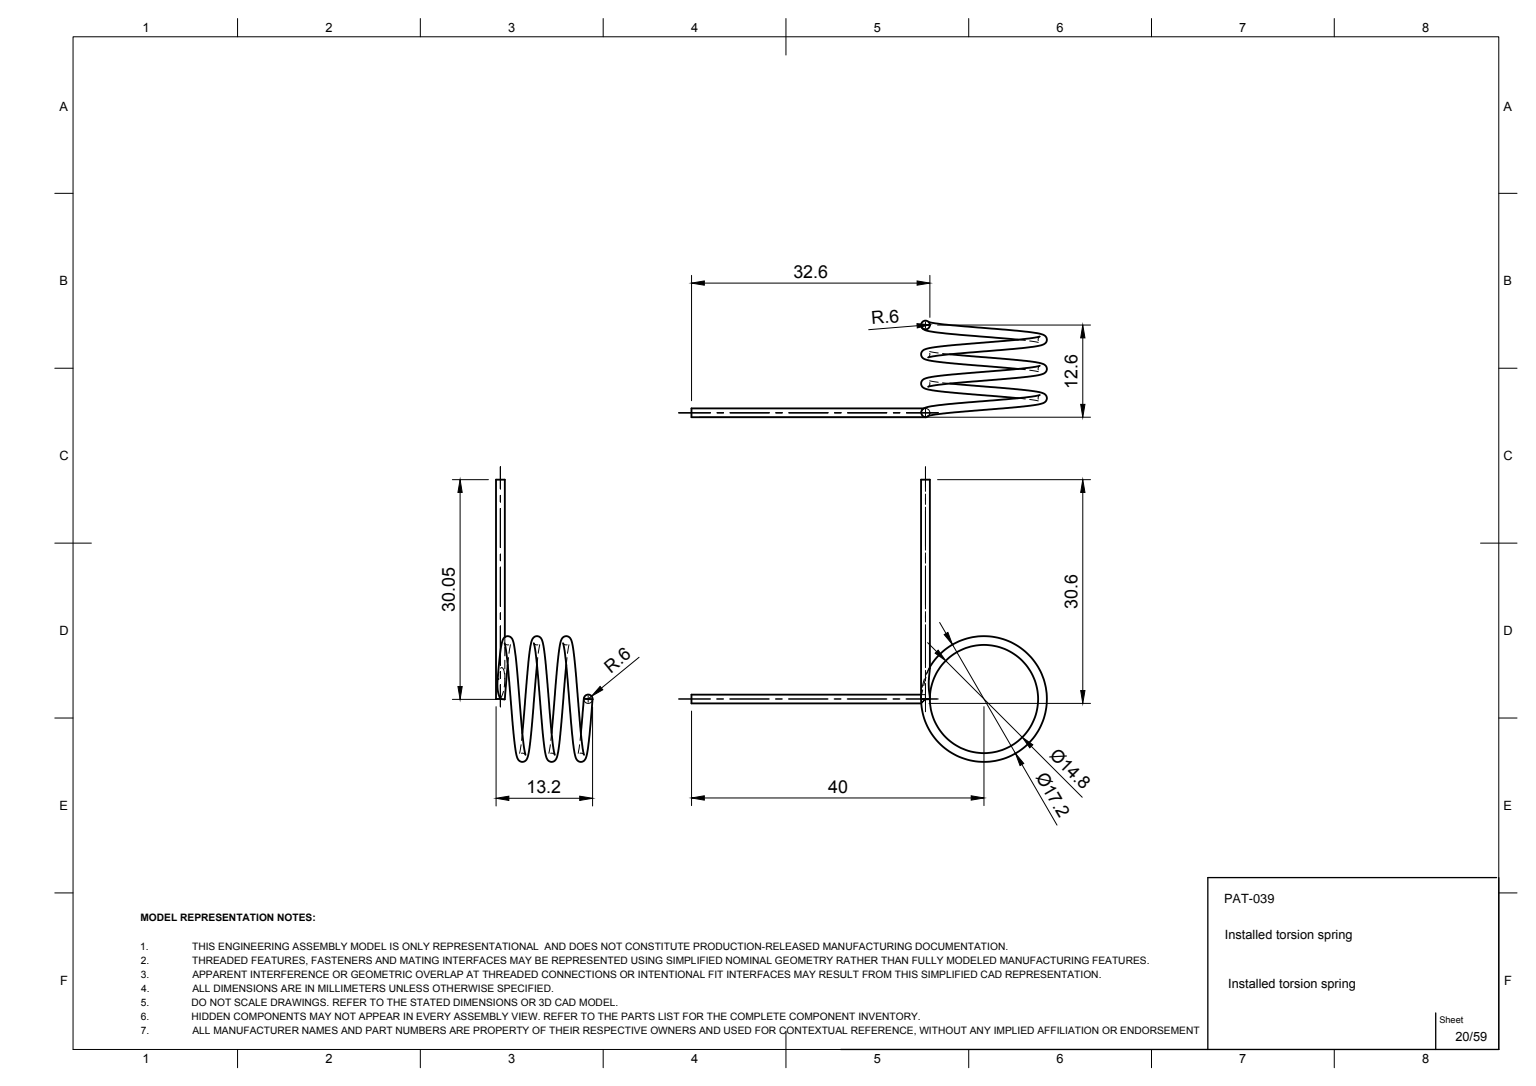
ISO-10303-21;
HEADER;
/* Generated by software containing ST-Developer
 * from STEP Tools, Inc. (www.steptools.com) 
 */

FILE_DESCRIPTION(
/* description */ ('Four-bar parallelogram arm'),
/* implementation_level */ '2;1');

FILE_NAME(
/* name */ 'Installed torsion spring.step',
/* time_stamp */ '2026-10-28T03:24:55-07:00',
/* author */ (''),
/* organization */ (''),
/* preprocessor_version */ 'ST-DEVELOPER v20.2',
/* originating_system */ 'Autodesk Translation Framework v15.17.0.0',
/* authorisation */ '');

FILE_SCHEMA (('AUTOMOTIVE_DESIGN { 1 0 10303 214 3 1 1 }'));
ENDSEC;

DATA;
#10=MECHANICAL_DESIGN_GEOMETRIC_PRESENTATION_REPRESENTATION('',(#637),#14512);
#497=B_SPLINE_SURFACE_WITH_KNOTS('',3,3,((#12064,#12065,#12066,#12067,#12068,
#12069,#12070,#12071,#12072,#12073,#12074,#12075,#12076,#12077,#12078,#12079,
#12080,#12081,#12082,#12083,#12084,#12085,#12086,#12087,#12088,#12089,#12090,
#12091,#12092,#12093,#12094,#12095,#12096,#12097,#12098,#12099,#12100,#12101,
#12102,#12103,#12104),(#12105,#12106,#12107,#12108,#12109,#12110,#12111,
#12112,#12113,#12114,#12115,#12116,#12117,#12118,#12119,#12120,#12121,#12122,
#12123,#12124,#12125,#12126,#12127,#12128,#12129,#12130,#12131,#12132,#12133,
#12134,#12135,#12136,#12137,#12138,#12139,#12140,#12141,#12142,#12143,#12144,
#12145),(#12146,#12147,#12148,#12149,#12150,#12151,#12152,#12153,#12154,
#12155,#12156,#12157,#12158,#12159,#12160,#12161,#12162,#12163,#12164,#12165,
#12166,#12167,#12168,#12169,#12170,#12171,#12172,#12173,#12174,#12175,#12176,
#12177,#12178,#12179,#12180,#12181,#12182,#12183,#12184,#12185,#12186),
(#12187,#12188,#12189,#12190,#12191,#12192,#12193,#12194,#12195,#12196,
#12197,#12198,#12199,#12200,#12201,#12202,#12203,#12204,#12205,#12206,#12207,
#12208,#12209,#12210,#12211,#12212,#12213,#12214,#12215,#12216,#12217,#12218,
#12219,#12220,#12221,#12222,#12223,#12224,#12225,#12226,#12227),(#12228,
#12229,#12230,#12231,#12232,#12233,#12234,#12235,#12236,#12237,#12238,#12239,
#12240,#12241,#12242,#12243,#12244,#12245,#12246,#12247,#12248,#12249,#12250,
#12251,#12252,#12253,#12254,#12255,#12256,#12257,#12258,#12259,#12260,#12261,
#12262,#12263,#12264,#12265,#12266,#12267,#12268),(#12269,#12270,#12271,
#12272,#12273,#12274,#12275,#12276,#12277,#12278,#12279,#12280,#12281,#12282,
#12283,#12284,#12285,#12286,#12287,#12288,#12289,#12290,#12291,#12292,#12293,
#12294,#12295,#12296,#12297,#12298,#12299,#12300,#12301,#12302,#12303,#12304,
#12305,#12306,#12307,#12308,#12309),(#12310,#12311,#12312,#12313,#12314,
#12315,#12316,#12317,#12318,#12319,#12320,#12321,#12322,#12323,#12324,#12325,
#12326,#12327,#12328,#12329,#12330,#12331,#12332,#12333,#12334,#12335,#12336,
#12337,#12338,#12339,#12340,#12341,#12342,#12343,#12344,#12345,#12346,#12347,
#12348,#12349,#12350),(#12351,#12352,#12353,#12354,#12355,#12356,#12357,
#12358,#12359,#12360,#12361,#12362,#12363,#12364,#12365,#12366,#12367,#12368,
#12369,#12370,#12371,#12372,#12373,#12374,#12375,#12376,#12377,#12378,#12379,
#12380,#12381,#12382,#12383,#12384,#12385,#12386,#12387,#12388,#12389,#12390,
#12391),(#12392,#12393,#12394,#12395,#12396,#12397,#12398,#12399,#12400,
#12401,#12402,#12403,#12404,#12405,#12406,#12407,#12408,#12409,#12410,#12411,
#12412,#12413,#12414,#12415,#12416,#12417,#12418,#12419,#12420,#12421,#12422,
#12423,#12424,#12425,#12426,#12427,#12428,#12429,#12430,#12431,#12432),
(#12433,#12434,#12435,#12436,#12437,#12438,#12439,#12440,#12441,#12442,
#12443,#12444,#12445,#12446,#12447,#12448,#12449,#12450,#12451,#12452,#12453,
#12454,#12455,#12456,#12457,#12458,#12459,#12460,#12461,#12462,#12463,#12464,
#12465,#12466,#12467,#12468,#12469,#12470,#12471,#12472,#12473)),
 .UNSPECIFIED.,.T.,.F.,.F.,(4,1,1,1,1,1,1,4),(4,1,1,1,1,1,1,1,1,1,1,1,1,
1,1,1,1,1,1,1,1,1,1,1,1,1,1,1,1,1,1,1,1,1,1,1,1,1,4),(-3.14159265358979,
-2.24399475256414,-1.34639685153848,-0.448798950512828,0.448798950512828,
1.34639685153848,2.24399475256414,3.14159265358979),(0.,0.0357142857142857,
0.0714285714285714,0.107142857142857,0.142857142857143,0.182539682539683,
0.19047619047619,0.214285714285714,0.238095238095238,0.261904761904762,
0.285714285714286,0.30952380952381,0.333333333333333,0.357142857142857,
0.380952380952381,0.412698412698413,0.420634920634921,0.428571428571429,
0.452380952380952,0.476190476190476,0.5,0.535714285714286,0.571428571428571,
0.607142857142857,0.642857142857143,0.678571428571428,0.696428571428571,
0.714285714285714,0.738095238095238,0.761904761904762,0.785714285714286,
0.809523809523809,0.833333333333333,0.857142857142857,0.875,0.892857142857143,
0.928571428571429,0.964285714285714,1.),.UNSPECIFIED.);
#498=B_SPLINE_CURVE_WITH_KNOTS('',3,(#11959,#11960,#11961,#11962,#11963,
#11964,#11965,#11966,#11967,#11968,#11969,#11970,#11971,#11972,#11973,#11974),
 .UNSPECIFIED.,.F.,.F.,(4,2,2,2,2,2,2,4),(-0.118162253960396,-0.11336417636029,
-0.0958062481624726,-0.0759366794145766,-0.0500215343183712,-0.0256788879713264,
0.,0.000489721640252749),.UNSPECIFIED.);
#499=B_SPLINE_CURVE_WITH_KNOTS('',3,(#11976,#11977,#11978,#11979,#11980,
#11981,#11982,#11983,#11984,#11985,#11986,#11987),.UNSPECIFIED.,.F.,.F.,
(4,2,2,2,2,4),(-0.218927972079618,-0.218528918486379,-0.18233291161771,
-0.153633681230302,-0.131619262867663,-0.118162253960396),.UNSPECIFIED.);
#500=B_SPLINE_CURVE_WITH_KNOTS('',3,(#12000,#12001,#12002,#12003,#12004,
#12005,#12006,#12007,#12008,#12009,#12010,#12011,#12012,#12013,#12014,#12015,
#12016,#12017,#12018,#12019,#12020,#12021,#12022,#12023,#12024,#12025,#12026,
#12027,#12028,#12029,#12030,#12031,#12032,#12033,#12034,#12035,#12036,#12037),
 .UNSPECIFIED.,.F.,.F.,(4,2,2,2,2,2,2,2,2,2,2,2,2,2,2,2,2,2,4),(-1.13171649654428,
-1.12635701987523,-0.945490005864125,-0.858292232112738,-0.829544128659967,
-0.817491257372727,-0.809719894883687,-0.801050781771893,-0.788842647214847,
-0.75932496601718,-0.695869882146734,-0.544122263235791,-0.475791925078994,
-0.456893383447211,-0.445776710112588,-0.436652368911013,-0.42698245595475,
-0.412387973442962,-0.410759286941866),.UNSPECIFIED.);
#501=B_SPLINE_CURVE_WITH_KNOTS('',3,(#12041,#12042,#12043,#12044,#12045,
#12046,#12047,#12048,#12049,#12050),.UNSPECIFIED.,.F.,.F.,(4,2,2,2,4),(-0.250413310593431,
-0.210654522228088,-0.0946898181455716,0.,0.00262144099416576),
 .UNSPECIFIED.);
#502=B_SPLINE_CURVE_WITH_KNOTS('',3,(#12051,#12052,#12053,#12054,#12055,
#12056,#12057,#12058),.UNSPECIFIED.,.F.,.F.,(4,2,2,4),(-0.410759286941866,
-0.382265373853863,-0.310503261016197,-0.250413310593431),.UNSPECIFIED.);
#503=B_SPLINE_CURVE_WITH_KNOTS('',3,(#12474,#12475,#12476,#12477,#12478,
#12479,#12480,#12481,#12482,#12483,#12484,#12485,#12486,#12487,#12488,#12489,
#12490,#12491,#12492,#12493,#12494,#12495,#12496,#12497,#12498,#12499,#12500,
#12501,#12502,#12503,#12504,#12505,#12506,#12507,#12508,#12509,#12510,#12511,
#12512,#12513,#12514,#12515,#12516,#12517,#12518,#12519,#12520,#12521,#12522,
#12523,#12524,#12525,#12526,#12527,#12528,#12529,#12530,#12531,#12532,#12533,
#12534,#12535,#12536,#12537,#12538,#12539,#12540,#12541,#12542,#12543,#12544,
#12545,#12546,#12547,#12548,#12549,#12550,#12551,#12552,#12553,#12554,#12555,
#12556,#12557,#12558,#12559,#12560,#12561,#12562,#12563,#12564,#12565,#12566,
#12567,#12568,#12569,#12570,#12571,#12572,#12573,#12574,#12575,#12576,#12577,
#12578,#12579,#12580,#12581,#12582,#12583,#12584,#12585,#12586,#12587,#12588),
 .UNSPECIFIED.,.F.,.F.,(4,3,3,3,3,3,3,3,3,3,3,3,3,3,3,3,3,3,3,3,3,3,3,3,
3,3,3,3,3,3,3,3,3,3,3,3,3,3,4),(0.0181496364157079,0.035714285714264,0.0714285714285062,
0.107142857142748,0.142857142856991,0.182539682539482,0.19047619047598,
0.214285714285475,0.23809523809497,0.261904761904465,0.28571428571396,0.309523809523454,
0.333333333332949,0.357142857142444,0.380952380951939,0.412698412697932,
0.42063492063443,0.428571428570928,0.452380952380423,0.476190476189918,
0.499999999999413,0.535714285713655,0.571428571427897,0.607142857142139,
0.642857142856382,0.678571428570624,0.696428571427745,0.714285714284866,
0.738095238094361,0.761904761903856,0.785714285713351,0.809523809522845,
0.83333333333234,0.857142857141835,0.874999999998956,0.892857142856077,
0.92857142857032,0.964285714284562,0.99631830509798),.UNSPECIFIED.);
#537=SHAPE_REPRESENTATION_RELATIONSHIP('SRR','None',#14758,#587);
#587=ADVANCED_BREP_SHAPE_REPRESENTATION('',(#695),#14473);
#637=STYLED_ITEM('',(#15087),#695);
#695=MANIFOLD_SOLID_BREP('Body1',#7341);
#1072=PLANE('',#8173);
#1073=PLANE('',#8174);
#1074=PLANE('',#8175);
#1075=PLANE('',#8180);
#1076=PLANE('',#8181);
#1077=PLANE('',#8182);
#1316=FACE_OUTER_BOUND('',#1807,.T.);
#1317=FACE_OUTER_BOUND('',#1808,.T.);
#1318=FACE_OUTER_BOUND('',#1809,.T.);
#1319=FACE_OUTER_BOUND('',#1810,.T.);
#1320=FACE_OUTER_BOUND('',#1811,.T.);
#1321=FACE_OUTER_BOUND('',#1812,.T.);
#1322=FACE_OUTER_BOUND('',#1813,.T.);
#1323=FACE_OUTER_BOUND('',#1814,.T.);
#1324=FACE_OUTER_BOUND('',#1815,.T.);
#1807=EDGE_LOOP('',(#5456,#5457,#5458,#5459,#5460,#5461,#5462));
#1808=EDGE_LOOP('',(#5463));
#1809=EDGE_LOOP('',(#5464,#5465,#5466));
#1810=EDGE_LOOP('',(#5467,#5468));
#1811=EDGE_LOOP('',(#5469,#5470,#5471,#5472,#5473,#5474,#5475));
#1812=EDGE_LOOP('',(#5476));
#1813=EDGE_LOOP('',(#5477,#5478));
#1814=EDGE_LOOP('',(#5479,#5480));
#1815=EDGE_LOOP('',(#5481,#5482,#5483,#5484,#5485,#5486,#5487,#5488,#5489));
#2448=LINE('',#11955,#2842);
#2449=LINE('',#11991,#2843);
#2450=LINE('',#11998,#2844);
#2451=LINE('',#12061,#2845);
#2842=VECTOR('',#9572,0.0599999999999996);
#2843=VECTOR('',#9581,1.);
#2844=VECTOR('',#9590,0.0600000000000001);
#2845=VECTOR('',#9597,1.);
#3198=CIRCLE('',#8170,0.0599999999999996);
#3199=CIRCLE('',#8171,0.0599999999999996);
#3200=CIRCLE('',#8172,0.0599999999999996);
#3201=CIRCLE('',#8176,0.06);
#3202=CIRCLE('',#8178,0.0600000000000001);
#3203=CIRCLE('',#8179,0.0600000000000001);
#3204=CIRCLE('',#8183,0.06);
#3701=VERTEX_POINT('',#11952);
#3702=VERTEX_POINT('',#11954);
#3703=VERTEX_POINT('',#11956);
#3704=VERTEX_POINT('',#11958);
#3705=VERTEX_POINT('',#11975);
#3706=VERTEX_POINT('',#11995);
#3707=VERTEX_POINT('',#11997);
#3708=VERTEX_POINT('',#11999);
#3709=VERTEX_POINT('',#12038);
#3710=VERTEX_POINT('',#12040);
#4359=EDGE_CURVE('',#3701,#3701,#3198,.T.);
#4360=EDGE_CURVE('',#3701,#3702,#2448,.T.);
#4361=EDGE_CURVE('',#3702,#3703,#3199,.T.);
#4362=EDGE_CURVE('',#3704,#3703,#498,.T.);
#4363=EDGE_CURVE('',#3705,#3704,#499,.T.);
#4364=EDGE_CURVE('',#3705,#3702,#3200,.T.);
#4365=EDGE_CURVE('',#3703,#3705,#2449,.T.);
#4366=EDGE_CURVE('',#3705,#3703,#3201,.T.);
#4367=EDGE_CURVE('',#3706,#3706,#3202,.T.);
#4368=EDGE_CURVE('',#3706,#3707,#2450,.T.);
#4369=EDGE_CURVE('',#3708,#3707,#500,.T.);
#4370=EDGE_CURVE('',#3708,#3709,#3203,.T.);
#4371=EDGE_CURVE('',#3710,#3709,#501,.T.);
#4372=EDGE_CURVE('',#3707,#3710,#502,.T.);
#4373=EDGE_CURVE('',#3709,#3708,#2451,.T.);
#4374=EDGE_CURVE('',#3709,#3708,#3204,.T.);
#4375=EDGE_CURVE('',#3710,#3704,#503,.T.);
#5456=ORIENTED_EDGE('',*,*,#4359,.F.);
#5457=ORIENTED_EDGE('',*,*,#4360,.T.);
#5458=ORIENTED_EDGE('',*,*,#4361,.T.);
#5459=ORIENTED_EDGE('',*,*,#4362,.F.);
#5460=ORIENTED_EDGE('',*,*,#4363,.F.);
#5461=ORIENTED_EDGE('',*,*,#4364,.T.);
#5462=ORIENTED_EDGE('',*,*,#4360,.F.);
#5463=ORIENTED_EDGE('',*,*,#4359,.T.);
#5464=ORIENTED_EDGE('',*,*,#4365,.F.);
#5465=ORIENTED_EDGE('',*,*,#4361,.F.);
#5466=ORIENTED_EDGE('',*,*,#4364,.F.);
#5467=ORIENTED_EDGE('',*,*,#4365,.T.);
#5468=ORIENTED_EDGE('',*,*,#4366,.T.);
#5469=ORIENTED_EDGE('',*,*,#4367,.F.);
#5470=ORIENTED_EDGE('',*,*,#4368,.T.);
#5471=ORIENTED_EDGE('',*,*,#4369,.F.);
#5472=ORIENTED_EDGE('',*,*,#4370,.T.);
#5473=ORIENTED_EDGE('',*,*,#4371,.F.);
#5474=ORIENTED_EDGE('',*,*,#4372,.F.);
#5475=ORIENTED_EDGE('',*,*,#4368,.F.);
#5476=ORIENTED_EDGE('',*,*,#4367,.T.);
#5477=ORIENTED_EDGE('',*,*,#4373,.F.);
#5478=ORIENTED_EDGE('',*,*,#4370,.F.);
#5479=ORIENTED_EDGE('',*,*,#4373,.T.);
#5480=ORIENTED_EDGE('',*,*,#4374,.F.);
#5481=ORIENTED_EDGE('',*,*,#4362,.T.);
#5482=ORIENTED_EDGE('',*,*,#4366,.F.);
#5483=ORIENTED_EDGE('',*,*,#4363,.T.);
#5484=ORIENTED_EDGE('',*,*,#4375,.F.);
#5485=ORIENTED_EDGE('',*,*,#4371,.T.);
#5486=ORIENTED_EDGE('',*,*,#4374,.T.);
#5487=ORIENTED_EDGE('',*,*,#4369,.T.);
#5488=ORIENTED_EDGE('',*,*,#4372,.T.);
#5489=ORIENTED_EDGE('',*,*,#4375,.T.);
#6763=CYLINDRICAL_SURFACE('',#8169,0.0599999999999996);
#6764=CYLINDRICAL_SURFACE('',#8177,0.0600000000000001);
#7021=ADVANCED_FACE('',(#1316),#6763,.T.);
#7022=ADVANCED_FACE('',(#1317),#1072,.T.);
#7023=ADVANCED_FACE('',(#1318),#1073,.F.);
#7024=ADVANCED_FACE('',(#1319),#1074,.T.);
#7025=ADVANCED_FACE('',(#1320),#6764,.T.);
#7026=ADVANCED_FACE('',(#1321),#1075,.T.);
#7027=ADVANCED_FACE('',(#1322),#1076,.F.);
#7028=ADVANCED_FACE('',(#1323),#1077,.F.);
#7029=ADVANCED_FACE('',(#1324),#497,.T.);
#7341=CLOSED_SHELL('',(#7021,#7022,#7023,#7024,#7025,#7026,#7027,#7028,
#7029));
#8168=AXIS2_PLACEMENT_3D('',#11950,#9566,#9567);
#8169=AXIS2_PLACEMENT_3D('',#11951,#9568,#9569);
#8170=AXIS2_PLACEMENT_3D('',#11953,#9570,#9571);
#8171=AXIS2_PLACEMENT_3D('',#11957,#9573,#9574);
#8172=AXIS2_PLACEMENT_3D('',#11988,#9575,#9576);
#8173=AXIS2_PLACEMENT_3D('',#11989,#9577,#9578);
#8174=AXIS2_PLACEMENT_3D('',#11990,#9579,#9580);
#8175=AXIS2_PLACEMENT_3D('',#11992,#9582,#9583);
#8176=AXIS2_PLACEMENT_3D('',#11993,#9584,#9585);
#8177=AXIS2_PLACEMENT_3D('',#11994,#9586,#9587);
#8178=AXIS2_PLACEMENT_3D('',#11996,#9588,#9589);
#8179=AXIS2_PLACEMENT_3D('',#12039,#9591,#9592);
#8180=AXIS2_PLACEMENT_3D('',#12059,#9593,#9594);
#8181=AXIS2_PLACEMENT_3D('',#12060,#9595,#9596);
#8182=AXIS2_PLACEMENT_3D('',#12062,#9598,#9599);
#8183=AXIS2_PLACEMENT_3D('',#12063,#9600,#9601);
#9566=DIRECTION('axis',(0.,0.,1.));
#9567=DIRECTION('refdir',(1.,0.,0.));
#9568=DIRECTION('center_axis',(1.,0.,0.));
#9569=DIRECTION('ref_axis',(0.,0.,-1.));
#9570=DIRECTION('center_axis',(1.,0.,0.));
#9571=DIRECTION('ref_axis',(0.,0.,-1.));
#9572=DIRECTION('',(-1.,0.,0.));
#9573=DIRECTION('center_axis',(1.,0.,0.));
#9574=DIRECTION('ref_axis',(0.,0.,-1.));
#9575=DIRECTION('center_axis',(1.,0.,0.));
#9576=DIRECTION('ref_axis',(0.,0.,-1.));
#9577=DIRECTION('center_axis',(1.,0.,0.));
#9578=DIRECTION('ref_axis',(0.,0.,-1.));
#9579=DIRECTION('center_axis',(1.,0.,0.));
#9580=DIRECTION('ref_axis',(0.,0.,-1.));
#9581=DIRECTION('',(0.,0.996867356793964,0.0790915479594076));
#9582=DIRECTION('center_axis',(0.000135869568084146,-0.0790915472293713,
0.99686734759261));
#9583=DIRECTION('ref_axis',(-0.997148648532906,-0.0752365903152447,-0.00583337010099326));
#9584=DIRECTION('center_axis',(0.000135869568084146,-0.0790915472293713,
0.99686734759261));
#9585=DIRECTION('ref_axis',(-0.997148648532906,-0.0752365903152447,-0.00583337010099326));
#9586=DIRECTION('center_axis',(0.,0.,1.));
#9587=DIRECTION('ref_axis',(1.,0.,0.));
#9588=DIRECTION('center_axis',(0.,0.,1.));
#9589=DIRECTION('ref_axis',(1.,0.,0.));
#9590=DIRECTION('',(0.,0.,-1.));
#9591=DIRECTION('center_axis',(0.,0.,1.));
#9592=DIRECTION('ref_axis',(1.,0.,0.));
#9593=DIRECTION('center_axis',(0.,0.,1.));
#9594=DIRECTION('ref_axis',(1.,0.,0.));
#9595=DIRECTION('center_axis',(0.,0.,1.));
#9596=DIRECTION('ref_axis',(1.,0.,0.));
#9597=DIRECTION('',(0.999998524451305,-0.00171787520298126,0.));
#9598=DIRECTION('center_axis',(-0.000135869608335795,-0.0790915472892204,
0.996867347587856));
#9599=DIRECTION('ref_axis',(1.07799071550222E-5,-0.996867356847137,-0.0790915465545881));
#9600=DIRECTION('center_axis',(-0.000135869608335795,-0.0790915472892204,
0.996867347587856));
#9601=DIRECTION('ref_axis',(1.07799071550222E-5,-0.996867356847137,-0.0790915465545882));
#11950=CARTESIAN_POINT('',(0.,0.,0.));
#11951=CARTESIAN_POINT('Origin',(0.8,-3.4,8.));
#11952=CARTESIAN_POINT('',(4.,-3.4,8.06));
#11953=CARTESIAN_POINT('Origin',(4.,-3.4,8.));
#11954=CARTESIAN_POINT('',(0.799999999999999,-3.4,8.06));
#11955=CARTESIAN_POINT('',(0.8,-3.4,8.06));
#11956=CARTESIAN_POINT('',(0.8,-3.45981204140764,7.99525450712245));
#11957=CARTESIAN_POINT('Origin',(0.8,-3.4,8.));
#11958=CARTESIAN_POINT('',(0.857757769669024,-3.39074044575272,7.94071880015435));
#11959=CARTESIAN_POINT('Ctrl Pts',(0.857757769669022,-3.39074044575271,
7.94071880015434));
#11960=CARTESIAN_POINT('Ctrl Pts',(0.857868134836737,-3.3922890292717,7.94047691582781));
#11961=CARTESIAN_POINT('Ctrl Pts',(0.857921908329668,-3.39385496848479,
7.94029447157442));
#11962=CARTESIAN_POINT('Ctrl Pts',(0.857899468660573,-3.401217652612,7.93973268518719));
#11963=CARTESIAN_POINT('Ctrl Pts',(0.857099131366584,-3.40693773045843,
7.94013905492094));
#11964=CARTESIAN_POINT('Ctrl Pts',(0.853922333121985,-3.41863574050482,
7.94261529275599));
#11965=CARTESIAN_POINT('Ctrl Pts',(0.851411692482855,-3.42433770210915,
7.94484920249294));
#11966=CARTESIAN_POINT('Ctrl Pts',(0.844348873784965,-3.43603698949541,
7.95142983480112));
#11967=CARTESIAN_POINT('Ctrl Pts',(0.83945370863678,-3.44153123637203,7.95616729134823));
#11968=CARTESIAN_POINT('Ctrl Pts',(0.829171203288947,-3.45001457070346,
7.96624704549874));
#11969=CARTESIAN_POINT('Ctrl Pts',(0.82379008497386,-3.45317277823043,7.97157628615011));
#11970=CARTESIAN_POINT('Ctrl Pts',(0.812442480882928,-3.45783692899872,
7.98285013462503));
#11971=CARTESIAN_POINT('Ctrl Pts',(0.80639623862599,-3.45926990278519,7.98887603141664));
#11972=CARTESIAN_POINT('Ctrl Pts',(0.800230800143543,-3.45979344585912,
7.9950243425463));
#11973=CARTESIAN_POINT('Ctrl Pts',(0.800115406102298,-3.45980291021815,
7.99513941790037));
#11974=CARTESIAN_POINT('Ctrl Pts',(0.799999999999999,-3.45981204140764,
7.99525450712243));
#11975=CARTESIAN_POINT('',(0.8,-3.34018795859236,8.00474549287757));
#11976=CARTESIAN_POINT('Ctrl Pts',(0.8,-3.34018795859236,8.00474549287757));
#11977=CARTESIAN_POINT('Ctrl Pts',(0.800115406079139,-3.3401788320092,8.00463046171348));
#11978=CARTESIAN_POINT('Ctrl Pts',(0.800230800092475,-3.34017003627816,
8.0045153917222));
#11979=CARTESIAN_POINT('Ctrl Pts',(0.810811727464239,-3.33939379801257,
7.99395951069901));
#11980=CARTESIAN_POINT('Ctrl Pts',(0.820900841739028,-3.34136574707449,
7.98346560010985));
#11981=CARTESIAN_POINT('Ctrl Pts',(0.836664447625529,-3.34957747484304,
7.96642056687488));
#11982=CARTESIAN_POINT('Ctrl Pts',(0.842584279376725,-3.35471818663018,
7.95976549836209));
#11983=CARTESIAN_POINT('Ctrl Pts',(0.850737922589237,-3.36590371591375,
7.95021852968304));
#11984=CARTESIAN_POINT('Ctrl Pts',(0.853638109640398,-3.37164357089127,
7.94665881249463));
#11985=CARTESIAN_POINT('Ctrl Pts',(0.856693627441668,-3.38219046561222,
7.94254333724378));
#11986=CARTESIAN_POINT('Ctrl Pts',(0.857448232148212,-3.38639718498341,
7.9413972050923));
#11987=CARTESIAN_POINT('Ctrl Pts',(0.857757769669022,-3.39074044575271,
7.94071880015434));
#11988=CARTESIAN_POINT('Origin',(0.8,-3.4,8.));
#11989=CARTESIAN_POINT('Origin',(4.,-3.4,8.));
#11990=CARTESIAN_POINT('Origin',(0.8,-3.4,8.));
#11991=CARTESIAN_POINT('',(0.8,-3.4,8.));
#11992=CARTESIAN_POINT('Origin',(0.8,-3.4,8.));
#11993=CARTESIAN_POINT('Origin',(0.8,-3.4,8.));
#11994=CARTESIAN_POINT('Origin',(0.8,-2.2,8.));
#11995=CARTESIAN_POINT('',(0.74,-2.2,11.));
#11996=CARTESIAN_POINT('Origin',(0.8,-2.2,11.));
#11997=CARTESIAN_POINT('',(0.739999999999999,-2.2,8.41884281581389));
#11998=CARTESIAN_POINT('',(0.74,-2.2,8.));
#11999=CARTESIAN_POINT('',(0.859999911467078,-2.20010307251212,8.));
#12000=CARTESIAN_POINT('Ctrl Pts',(0.859999911467078,-2.20010307251221,
8.));
#12001=CARTESIAN_POINT('Ctrl Pts',(0.859999136901991,-2.20055395738578,
8.00090497885833));
#12002=CARTESIAN_POINT('Ctrl Pts',(0.859993279965474,-2.20100479566276,
8.00180978698512));
#12003=CARTESIAN_POINT('Ctrl Pts',(0.859613264338125,-2.21666553404949,
8.03325602937855));
#12004=CARTESIAN_POINT('Ctrl Pts',(0.853474853505761,-2.23105407285076,
8.06256859999788));
#12005=CARTESIAN_POINT('Ctrl Pts',(0.838027444543347,-2.24696762823943,
8.12558745018579));
#12006=CARTESIAN_POINT('Ctrl Pts',(0.832681318070563,-2.25065802014274,
8.14673824214296));
#12007=CARTESIAN_POINT('Ctrl Pts',(0.825757894768706,-2.25422415942331,
8.17441882347885));
#12008=CARTESIAN_POINT('Ctrl Pts',(0.824032187048781,-2.25500826562799,
8.18131842676915));
#12009=CARTESIAN_POINT('Ctrl Pts',(0.821583106170439,-2.25598907832281,
8.1910847498449));
#12010=CARTESIAN_POINT('Ctrl Pts',(0.820858026692738,-2.25626310384707,
8.19397291910405));
#12011=CARTESIAN_POINT('Ctrl Pts',(0.819663731786288,-2.2566884878246,8.19872186244263));
#12012=CARTESIAN_POINT('Ctrl Pts',(0.819194803735207,-2.25684895568773,
8.20058440860189));
#12013=CARTESIAN_POINT('Ctrl Pts',(0.818201492584122,-2.25717525350113,
8.20452431789242));
#12014=CARTESIAN_POINT('Ctrl Pts',(0.817676638293826,-2.25733966745791,
8.20660292114951));
#12015=CARTESIAN_POINT('Ctrl Pts',(0.816410515141555,-2.25771734508197,
8.2116077883401));
#12016=CARTESIAN_POINT('Ctrl Pts',(0.815667569715253,-2.25792338856219,
8.21453683995452));
#12017=CARTESIAN_POINT('Ctrl Pts',(0.813121121086004,-2.25857725854118,
8.22454278593531));
#12018=CARTESIAN_POINT('Ctrl Pts',(0.811298366698271,-2.25895601380967,
8.23164788351326));
#12019=CARTESIAN_POINT('Ctrl Pts',(0.805508922328413,-2.25988040695531,
8.25394436711295));
#12020=CARTESIAN_POINT('Ctrl Pts',(0.801392906371853,-2.26013248433115,
8.26939428603274));
#12021=CARTESIAN_POINT('Ctrl Pts',(0.787077992513295,-2.25945702001813,
8.32085142392661));
#12022=CARTESIAN_POINT('Ctrl Pts',(0.777263862165306,-2.25647828649788,
8.35220541029103));
#12023=CARTESIAN_POINT('Ctrl Pts',(0.764515912500924,-2.24860576017211,
8.38771594041925));
#12024=CARTESIAN_POINT('Ctrl Pts',(0.757692854619132,-2.24378973207509,
8.40584390296175));
#12025=CARTESIAN_POINT('Ctrl Pts',(0.749880792752036,-2.23311016839464,
8.42116977302821));
#12026=CARTESIAN_POINT('Ctrl Pts',(0.748053813348503,-2.23026329396527,
8.42439613938683));
#12027=CARTESIAN_POINT('Ctrl Pts',(0.74536508490224,-2.22489909228887,8.42792153395599));
#12028=CARTESIAN_POINT('Ctrl Pts',(0.74440239044637,-2.22270189648639,8.42889596208619));
#12029=CARTESIAN_POINT('Ctrl Pts',(0.742834762688225,-2.2183437876705,8.42963752815454));
#12030=CARTESIAN_POINT('Ctrl Pts',(0.742234963015787,-2.21635394379078,
8.42957119646972));
#12031=CARTESIAN_POINT('Ctrl Pts',(0.741219113742224,-2.21223036963063,
8.42860540961881));
#12032=CARTESIAN_POINT('Ctrl Pts',(0.740845869213951,-2.21021743019184,
8.42768512388005));
#12033=CARTESIAN_POINT('Ctrl Pts',(0.740183709016934,-2.20549798416793,
8.42469682244956));
#12034=CARTESIAN_POINT('Ctrl Pts',(0.740031560493762,-2.20294644611918,
8.42227427643572));
#12035=CARTESIAN_POINT('Ctrl Pts',(0.740001469953493,-2.20048719247971,
8.419426543521));
#12036=CARTESIAN_POINT('Ctrl Pts',(0.739999999999999,-2.20024249519991,
8.41913657657253));
#12037=CARTESIAN_POINT('Ctrl Pts',(0.739999999999999,-2.2,8.41884281581389));
#12038=CARTESIAN_POINT('',(0.740000088532922,-2.19989692748782,8.));
#12039=CARTESIAN_POINT('Origin',(0.8,-2.2,8.));
#12040=CARTESIAN_POINT('',(0.753574871202513,-2.16199069301438,8.27341677618955));
#12041=CARTESIAN_POINT('Ctrl Pts',(0.753574871223386,-2.16199069300718,
8.2734167761916));
#12042=CARTESIAN_POINT('Ctrl Pts',(0.754683939292676,-2.16063606089172,
8.25732450111787));
#12043=CARTESIAN_POINT('Ctrl Pts',(0.755525382712852,-2.15972125718946,
8.24070221271168));
#12044=CARTESIAN_POINT('Ctrl Pts',(0.757139618224984,-2.15797471815607,
8.17493064758107));
#12045=CARTESIAN_POINT('Ctrl Pts',(0.753939881287673,-2.16024262281511,
8.13023220048983));
#12046=CARTESIAN_POINT('Ctrl Pts',(0.744417566034987,-2.17594334474188,
8.05631746291443));
#12047=CARTESIAN_POINT('Ctrl Pts',(0.740253147200178,-2.18623233338143,
8.03133361374068));
#12048=CARTESIAN_POINT('Ctrl Pts',(0.740004341424627,-2.19919813034124,
8.00160163133619));
#12049=CARTESIAN_POINT('Ctrl Pts',(0.74000068880078,-2.19954750340221,8.00080090746578));
#12050=CARTESIAN_POINT('Ctrl Pts',(0.740000088532922,-2.19989692748782,
8.));
#12051=CARTESIAN_POINT('Ctrl Pts',(0.739999999999999,-2.2,8.41884281581389));
#12052=CARTESIAN_POINT('Ctrl Pts',(0.739999999999998,-2.19575754011241,
8.41370346363053));
#12053=CARTESIAN_POINT('Ctrl Pts',(0.740440387962112,-2.19219010800851,
8.40740207004508));
#12054=CARTESIAN_POINT('Ctrl Pts',(0.742244557849095,-2.18218933179936,
8.38643590161123));
#12055=CARTESIAN_POINT('Ctrl Pts',(0.74470820844627,-2.17604859945841,8.366170220377));
#12056=CARTESIAN_POINT('Ctrl Pts',(0.749610729583609,-2.16709782252209,
8.32084795754587));
#12057=CARTESIAN_POINT('Ctrl Pts',(0.751898667092447,-2.16403803348222,
8.29773804077552));
#12058=CARTESIAN_POINT('Ctrl Pts',(0.753574871223386,-2.16199069300717,
8.2734167761916));
#12059=CARTESIAN_POINT('Origin',(0.8,-2.2,11.));
#12060=CARTESIAN_POINT('Origin',(0.8,-2.2,8.));
#12061=CARTESIAN_POINT('',(0.8,-2.2,8.));
#12062=CARTESIAN_POINT('Origin',(0.8,-2.2,8.));
#12063=CARTESIAN_POINT('Origin',(0.8,-2.2,8.));
#12064=CARTESIAN_POINT('Ctrl Pts',(0.799999353205571,-2.14018795858917,
8.00474549279328));
#12065=CARTESIAN_POINT('Ctrl Pts',(0.799974799734663,-2.15448086801293,
8.18489286877592));
#12066=CARTESIAN_POINT('Ctrl Pts',(0.674665007466417,-2.18310389914977,
8.54360793631645));
#12067=CARTESIAN_POINT('Ctrl Pts',(0.189057319427946,-2.22621797906703,
8.84931316013818));
#12068=CARTESIAN_POINT('Ctrl Pts',(-0.382526459311769,-2.26949883233014,
8.78512361823764));
#12069=CARTESIAN_POINT('Ctrl Pts',(-0.807840639236961,-2.31455899583364,
8.36128354752488));
#12070=CARTESIAN_POINT('Ctrl Pts',(-0.841884630553248,-2.34849059789531,
7.90616153590567));
#12071=CARTESIAN_POINT('Ctrl Pts',(-0.706633312481697,-2.3776482221266,
7.56417102566761));
#12072=CARTESIAN_POINT('Ctrl Pts',(-0.524797421299121,-2.40036397277687,
7.33517763260607));
#12073=CARTESIAN_POINT('Ctrl Pts',(-0.184623097405697,-2.42964203470304,
7.17129916558269));
#12074=CARTESIAN_POINT('Ctrl Pts',(0.193484153574259,-2.4589910981866,7.17122122775637));
#12075=CARTESIAN_POINT('Ctrl Pts',(0.53519122257586,-2.48841027946974,7.33563982396839));
#12076=CARTESIAN_POINT('Ctrl Pts',(0.772150285550503,-2.51789845810207,
7.63264106317873));
#12077=CARTESIAN_POINT('Ctrl Pts',(0.857109363647141,-2.54745448449862,
8.00408762003218));
#12078=CARTESIAN_POINT('Ctrl Pts',(0.772052203859602,-2.5770771143395,8.37600483173473));
#12079=CARTESIAN_POINT('Ctrl Pts',(0.507269008134946,-2.61006365580992,
8.70902087610833));
#12080=CARTESIAN_POINT('Ctrl Pts',(0.184121132841334,-2.63651910824196,
8.83624322508014));
#12081=CARTESIAN_POINT('Ctrl Pts',(-0.066489483803979,-2.65639505342702,
8.83575881359142));
#12082=CARTESIAN_POINT('Ctrl Pts',(-0.272993262404685,-2.67296969383809,
8.80486180272118));
#12083=CARTESIAN_POINT('Ctrl Pts',(-0.542963798600168,-2.69620569938568,
8.6749478571166));
#12084=CARTESIAN_POINT('Ctrl Pts',(-0.783400610994973,-2.72613969346878,
8.3735180635455));
#12085=CARTESIAN_POINT('Ctrl Pts',(-0.884539863210645,-2.76112964475965,
7.93383176138089));
#12086=CARTESIAN_POINT('Ctrl Pts',(-0.709496036003296,-2.80121083689286,
7.43066574821048));
#12087=CARTESIAN_POINT('Ctrl Pts',(-0.200096069822599,-2.84642092016874,
7.11042023888795));
#12088=CARTESIAN_POINT('Ctrl Pts',(0.398680163779428,-2.89174303462223,
7.17762409038781));
#12089=CARTESIAN_POINT('Ctrl Pts',(0.826194257186495,-2.93717015873569,
7.60494403903258));
#12090=CARTESIAN_POINT('Ctrl Pts',(0.883028763967666,-2.97510749619044,
8.10591734828594));
#12091=CARTESIAN_POINT('Ctrl Pts',(0.733685094600885,-3.00550240345549,
8.46374186218363));
#12092=CARTESIAN_POINT('Ctrl Pts',(0.518762431301621,-3.03085542203816,
8.70482943573385));
#12093=CARTESIAN_POINT('Ctrl Pts',(0.194479876070813,-3.05877306117867,
8.86101946641206));
#12094=CARTESIAN_POINT('Ctrl Pts',(-0.198398854087579,-3.08926279897463,
8.86116295997746));
#12095=CARTESIAN_POINT('Ctrl Pts',(-0.552866770740287,-3.11978430147565,
8.69045288806385));
#12096=CARTESIAN_POINT('Ctrl Pts',(-0.798459570530803,-3.15033499607393,
8.38276097552609));
#12097=CARTESIAN_POINT('Ctrl Pts',(-0.886189886223361,-3.18091257250085,
7.9985222617957));
#12098=CARTESIAN_POINT('Ctrl Pts',(-0.805754444707439,-3.20896404488721,
7.64600910454789));
#12099=CARTESIAN_POINT('Ctrl Pts',(-0.617356025266483,-3.23448146889928,
7.38101130632405));
#12100=CARTESIAN_POINT('Ctrl Pts',(-0.299249903140631,-3.2651162608211,
7.15427322620025));
#12101=CARTESIAN_POINT('Ctrl Pts',(0.20669102063405,-3.30343842772452,7.09641469177514));
#12102=CARTESIAN_POINT('Ctrl Pts',(0.72520383869486,-3.34944736574065,7.4225450742071));
#12103=CARTESIAN_POINT('Ctrl Pts',(0.859802571238952,-3.38014846116659,
7.80703861326121));
#12104=CARTESIAN_POINT('Ctrl Pts',(0.859828918911975,-3.39548580458109,
8.00035000220606));
#12105=CARTESIAN_POINT('Ctrl Pts',(0.782047395351802,-2.14018795858917,
8.00474304600285));
#12106=CARTESIAN_POINT('Ctrl Pts',(0.782023383332822,-2.15416568148035,
8.18091782094919));
#12107=CARTESIAN_POINT('Ctrl Pts',(0.659521780500366,-2.18214688322478,
8.53162368091412));
#12108=CARTESIAN_POINT('Ctrl Pts',(0.18464317703468,-2.22430909576203,8.83062018723366));
#12109=CARTESIAN_POINT('Ctrl Pts',(-0.374447713497299,-2.26664059058254,
8.76785144918027));
#12110=CARTESIAN_POINT('Ctrl Pts',(-0.790610270786435,-2.31072617143467,
8.35318712238713));
#12111=CARTESIAN_POINT('Ctrl Pts',(-0.823965551575852,-2.34393500774394,
7.90772402533263));
#12112=CARTESIAN_POINT('Ctrl Pts',(-0.69154722527925,-2.37248233285328,
7.57288615600467));
#12113=CARTESIAN_POINT('Ctrl Pts',(-0.513499356518822,-2.3947239401174,
7.34864384720008));
#12114=CARTESIAN_POINT('Ctrl Pts',(-0.18028811648245,-2.4234026384316,7.18809946898689));
#12115=CARTESIAN_POINT('Ctrl Pts',(0.190198277819923,-2.45215741125776,
7.18800542247321));
#12116=CARTESIAN_POINT('Ctrl Pts',(0.525149537887764,-2.48099201036255,
7.34914925604369));
#12117=CARTESIAN_POINT('Ctrl Pts',(0.757517539664766,-2.50990501139262,
7.64036832969054));
#12118=CARTESIAN_POINT('Ctrl Pts',(0.840880626162148,-2.53889479412451,
8.00473123017728));
#12119=CARTESIAN_POINT('Ctrl Pts',(0.757422383748918,-2.56796498202542,
8.36973245506803));
#12120=CARTESIAN_POINT('Ctrl Pts',(0.497481478898117,-2.60034773025975,
8.69669786914853));
#12121=CARTESIAN_POINT('Ctrl Pts',(0.180051704651674,-2.62633437324586,
8.82170336201811));
#12122=CARTESIAN_POINT('Ctrl Pts',(-0.0662397268939709,-2.64586682880387,
8.8212287792569));
#12123=CARTESIAN_POINT('Ctrl Pts',(-0.269218207817606,-2.66215808538477,
8.79086083019633));
#12124=CARTESIAN_POINT('Ctrl Pts',(-0.534658210265181,-2.68500042855823,
8.66314528058294));
#12125=CARTESIAN_POINT('Ctrl Pts',(-0.77121061187554,-2.71444724443111,
8.36662469936537));
#12126=CARTESIAN_POINT('Ctrl Pts',(-0.870785710837989,-2.74888478105817,
7.93385634133438));
#12127=CARTESIAN_POINT('Ctrl Pts',(-0.698451578107866,-2.78835482764175,
7.43825459451075));
#12128=CARTESIAN_POINT('Ctrl Pts',(-0.196333892591823,-2.83291723989608,
7.12247712438595));
#12129=CARTESIAN_POINT('Ctrl Pts',(0.394483807013738,-2.87762888342211,
7.18869373683052));
#12130=CARTESIAN_POINT('Ctrl Pts',(0.81676492629728,-2.92248617467578,7.61064729804906));
#12131=CARTESIAN_POINT('Ctrl Pts',(0.87303850287666,-2.95998625249499,8.10588405657973));
#12132=CARTESIAN_POINT('Ctrl Pts',(0.725307987087691,-2.99005251598402,
8.45988987866063));
#12133=CARTESIAN_POINT('Ctrl Pts',(0.512589152625104,-3.0151452729584,8.69852906415756));
#12134=CARTESIAN_POINT('Ctrl Pts',(0.191449002788501,-3.04278955011802,
8.85323712338039));
#12135=CARTESIAN_POINT('Ctrl Pts',(-0.197922943695345,-3.07300561720271,
8.85341423236731));
#12136=CARTESIAN_POINT('Ctrl Pts',(-0.549461136454415,-3.10326898677065,
8.68414590340907));
#12137=CARTESIAN_POINT('Ctrl Pts',(-0.793229818870514,-3.13358792502119,
8.37879861499031));
#12138=CARTESIAN_POINT('Ctrl Pts',(-0.880383072820295,-3.1639499541908,
7.99721589789444));
#12139=CARTESIAN_POINT('Ctrl Pts',(-0.800475324765631,-3.1918254698827,
7.64687170048445));
#12140=CARTESIAN_POINT('Ctrl Pts',(-0.61312934238898,-3.21719954694791,
7.38332949897577));
#12141=CARTESIAN_POINT('Ctrl Pts',(-0.296622142271461,-3.24767997051828,
7.15770725112751));
#12142=CARTESIAN_POINT('Ctrl Pts',(0.207147409687023,-3.28583242893591,
7.10000791688759));
#12143=CARTESIAN_POINT('Ctrl Pts',(0.724104113244679,-3.33169443325757,
7.42503466252389));
#12144=CARTESIAN_POINT('Ctrl Pts',(0.858447915360046,-3.36232685262669,
7.80874538280109));
#12145=CARTESIAN_POINT('Ctrl Pts',(0.858474223399892,-3.37764112502309,
8.00176598536707));
#12146=CARTESIAN_POINT('Ctrl Pts',(0.74625274599145,-2.15732833022565,8.00337824864829));
#12147=CARTESIAN_POINT('Ctrl Pts',(0.746229817884691,-2.17067509306803,
8.17160042319879));
#12148=CARTESIAN_POINT('Ctrl Pts',(0.629314000947051,-2.19736550953753,
8.50610935856775));
#12149=CARTESIAN_POINT('Ctrl Pts',(0.176611094607005,-2.23755733973025,
8.79107825953155));
#12150=CARTESIAN_POINT('Ctrl Pts',(-0.355910946191055,-2.27787674797685,
8.73120669874899));
#12151=CARTESIAN_POINT('Ctrl Pts',(-0.752030415880074,-2.31984419599776,
8.33643709393526));
#12152=CARTESIAN_POINT('Ctrl Pts',(-0.783731715249715,-2.35144232472123,
7.91257415253098));
#12153=CARTESIAN_POINT('Ctrl Pts',(-0.657760402987585,-2.37859990065862,
7.59404159903955));
#12154=CARTESIAN_POINT('Ctrl Pts',(-0.488391328153346,-2.3997571052949,
7.38074179934443));
#12155=CARTESIAN_POINT('Ctrl Pts',(-0.17146818986477,-2.42703420947409,
7.22805123116321));
#12156=CARTESIAN_POINT('Ctrl Pts',(0.180899194564967,-2.45438379948815,
7.22796563928441));
#12157=CARTESIAN_POINT('Ctrl Pts',(0.499476525914112,-2.48181004852974,
7.38123478608588));
#12158=CARTESIAN_POINT('Ctrl Pts',(0.720509655667483,-2.50931350242048,
7.65824455912636));
#12159=CARTESIAN_POINT('Ctrl Pts',(0.799820849374384,-2.53689527427906,
8.00488898306531));
#12160=CARTESIAN_POINT('Ctrl Pts',(0.720413518964486,-2.56455811211287,
8.35221369057467));
#12161=CARTESIAN_POINT('Ctrl Pts',(0.472996082608528,-2.59538372533697,
8.66344434480147));
#12162=CARTESIAN_POINT('Ctrl Pts',(0.170739321333303,-2.62012995691034,
8.78249789645164));
#12163=CARTESIAN_POINT('Ctrl Pts',(-0.0638674325015451,-2.63873618276797,
8.78204801163947));
#12164=CARTESIAN_POINT('Ctrl Pts',(-0.257241904787735,-2.65425698108223,
8.75311696166082));
#12165=CARTESIAN_POINT('Ctrl Pts',(-0.510220632940824,-2.67602856460628,
8.63141433807984));
#12166=CARTESIAN_POINT('Ctrl Pts',(-0.735784166111144,-2.70410650625065,
8.34869879134964));
#12167=CARTESIAN_POINT('Ctrl Pts',(-0.830811311210507,-2.73696323384205,
7.9358300220051));
#12168=CARTESIAN_POINT('Ctrl Pts',(-0.666338844974052,-2.77465593116664,
7.46259060542153));
#12169=CARTESIAN_POINT('Ctrl Pts',(-0.186452486819304,-2.81725520701278,
7.16066959619675));
#12170=CARTESIAN_POINT('Ctrl Pts',(0.378959513489126,-2.86004954464569,
7.2239233219175));
#12171=CARTESIAN_POINT('Ctrl Pts',(0.783699385156277,-2.90303928187437,
7.62816364103489));
#12172=CARTESIAN_POINT('Ctrl Pts',(0.837802742196778,-2.9390268509025,8.10336709497288));
#12173=CARTESIAN_POINT('Ctrl Pts',(0.695903933635387,-2.96791382473259,
8.44346809432988));
#12174=CARTESIAN_POINT('Ctrl Pts',(0.491405830641922,-2.99204008047502,
8.67290813935407));
#12175=CARTESIAN_POINT('Ctrl Pts',(0.18237238112984,-3.01864752247096,8.82183051955883));
#12176=CARTESIAN_POINT('Ctrl Pts',(-0.192742934390733,-3.04775885609569,
8.82204356332466));
#12177=CARTESIAN_POINT('Ctrl Pts',(-0.531846282469671,-3.07695455750375,
8.65882083669825));
#12178=CARTESIAN_POINT('Ctrl Pts',(-0.767277470964291,-3.1062336310193,
8.36398870428271));
#12179=CARTESIAN_POINT('Ctrl Pts',(-0.851599932176543,-3.1355956353591,
7.99504782175763));
#12180=CARTESIAN_POINT('Ctrl Pts',(-0.774285320211519,-3.16258542373216,
7.65586242334073));
#12181=CARTESIAN_POINT('Ctrl Pts',(-0.592726533508006,-3.18718054137099,
7.40042073906037));
#12182=CARTESIAN_POINT('Ctrl Pts',(-0.285687289089679,-3.2167534027861,
7.18150928308508));
#12183=CARTESIAN_POINT('Ctrl Pts',(0.203822077518427,-3.2538348995878,7.12528061883726));
#12184=CARTESIAN_POINT('Ctrl Pts',(0.707318122939241,-3.2984956193622,7.44157309236475));
#12185=CARTESIAN_POINT('Ctrl Pts',(0.838602160088046,-3.32839609386495,
7.81596220818301));
#12186=CARTESIAN_POINT('Ctrl Pts',(0.838627855643513,-3.34335383066725,
8.0044890474524));
#12187=CARTESIAN_POINT('Ctrl Pts',(0.733109166050823,-2.21520789437687,
7.99878428726588));
#12188=CARTESIAN_POINT('Ctrl Pts',(0.733086651152081,-2.22831412321213,
8.16397477883759));
#12189=CARTESIAN_POINT('Ctrl Pts',(0.61820806476396,-2.25448891667089,8.4918749804416));
#12190=CARTESIAN_POINT('Ctrl Pts',(0.175997071981037,-2.2937344485149,8.76979482863797));
#12191=CARTESIAN_POINT('Ctrl Pts',(-0.341851058364153,-2.33295097190823,
8.71124005417684));
#12192=CARTESIAN_POINT('Ctrl Pts',(-0.725322381060742,-2.37361034528651,
8.3285616317421));
#12193=CARTESIAN_POINT('Ctrl Pts',(-0.755620395377764,-2.40410249010971,
7.91958143791062));
#12194=CARTESIAN_POINT('Ctrl Pts',(-0.634368791517699,-2.43024050309635,
7.61303100221757));
#12195=CARTESIAN_POINT('Ctrl Pts',(-0.471556266419422,-2.45057518839065,
7.40809066379694));
#12196=CARTESIAN_POINT('Ctrl Pts',(-0.167691580481213,-2.4767255191272,
7.26180006781177));
#12197=CARTESIAN_POINT('Ctrl Pts',(0.169354507378634,-2.50288963142343,
7.26180070426125));
#12198=CARTESIAN_POINT('Ctrl Pts',(0.473364185136383,-2.52906730718321,
7.40815784881158));
#12199=CARTESIAN_POINT('Ctrl Pts',(0.683803616304868,-2.555262600058,7.67201422540797));
#12200=CARTESIAN_POINT('Ctrl Pts',(0.759102306253096,-2.58147909308525,
8.00147874603806));
#12201=CARTESIAN_POINT('Ctrl Pts',(0.683721893443959,-2.60771728231028,
8.33088235794537));
#12202=CARTESIAN_POINT('Ctrl Pts',(0.449432489049715,-2.63690187004837,
8.62546727981126));
#12203=CARTESIAN_POINT('Ctrl Pts',(0.163874330576686,-2.66027910711593,
8.73783282899925));
#12204=CARTESIAN_POINT('Ctrl Pts',(-0.0574129106102927,-2.6778300800841,
8.73740397568539));
#12205=CARTESIAN_POINT('Ctrl Pts',(-0.239710347551256,-2.69246200371179,
8.71012676650314));
#12206=CARTESIAN_POINT('Ctrl Pts',(-0.47792311168767,-2.71296689041938,
8.59547666875305));
#12207=CARTESIAN_POINT('Ctrl Pts',(-0.689948244038352,-2.73936587099675,
8.32963733232912));
#12208=CARTESIAN_POINT('Ctrl Pts',(-0.779095823746774,-2.77021281732857,
7.94202402152301));
#12209=CARTESIAN_POINT('Ctrl Pts',(-0.62481378813293,-2.80554090335429,
7.49856445460143));
#12210=CARTESIAN_POINT('Ctrl Pts',(-0.175855711648067,-2.84539012232819,
7.21629185933956));
#12211=CARTESIAN_POINT('Ctrl Pts',(0.352109156831138,-2.88535475052917,
7.27549305282249));
#12212=CARTESIAN_POINT('Ctrl Pts',(0.72941562263406,-2.92544247381862,7.65250150966383));
#12213=CARTESIAN_POINT('Ctrl Pts',(0.779714856881808,-2.9589572593585,8.09504757135279));
#12214=CARTESIAN_POINT('Ctrl Pts',(0.647663516769697,-2.98583864019596,
8.41151349407204));
#12215=CARTESIAN_POINT('Ctrl Pts',(0.45745146394856,-3.00827891026592,8.62491004682719));
#12216=CARTESIAN_POINT('Ctrl Pts',(0.170146416399821,-3.03301596259707,
8.7633430911453));
#12217=CARTESIAN_POINT('Ctrl Pts',(-0.178425509553831,-3.06006759257889,
8.76352533431625));
#12218=CARTESIAN_POINT('Ctrl Pts',(-0.493423394438939,-3.08718913671925,
8.61189555627018));
#12219=CARTESIAN_POINT('Ctrl Pts',(-0.712056882382278,-3.1143800682777,
8.33808617234675));
#12220=CARTESIAN_POINT('Ctrl Pts',(-0.790352964968391,-3.14164438601587,
7.99550913276558));
#12221=CARTESIAN_POINT('Ctrl Pts',(-0.718569670978983,-3.16670409444998,
7.68058308222211));
#12222=CARTESIAN_POINT('Ctrl Pts',(-0.549995050890336,-3.18954068246379,
7.44339985556457));
#12223=CARTESIAN_POINT('Ctrl Pts',(-0.264888955600131,-3.21700180066857,
7.2401273936459));
#12224=CARTESIAN_POINT('Ctrl Pts',(0.18973412922727,-3.25143927114534,7.18784224870088));
#12225=CARTESIAN_POINT('Ctrl Pts',(0.657612957996916,-3.29294170706199,
7.48173687430083));
#12226=CARTESIAN_POINT('Ctrl Pts',(0.779716152438242,-3.3207351361234,7.8297224617271));
#12227=CARTESIAN_POINT('Ctrl Pts',(0.779740067663557,-3.33465651822015,
8.00518711922511));
#12228=CARTESIAN_POINT('Ctrl Pts',(0.770174713816319,-2.26178036861328,
7.99509427477235));
#12229=CARTESIAN_POINT('Ctrl Pts',(0.770151085712947,-2.27553460900681,
8.16845228342319));
#12230=CARTESIAN_POINT('Ctrl Pts',(0.649526282375535,-2.30298809044055,
8.51236935836145));
#12231=CARTESIAN_POINT('Ctrl Pts',(0.187191988159535,-2.34399875981116,
8.80253374467715));
#12232=CARTESIAN_POINT('Ctrl Pts',(-0.352122720593585,-2.38484196589621,
8.74127014025205));
#12233=CARTESIAN_POINT('Ctrl Pts',(-0.74981389952082,-2.42703190005934,
8.34386831568528));
#12234=CARTESIAN_POINT('Ctrl Pts',(-0.780810988575083,-2.45854730667668,
7.92110588453579));
#12235=CARTESIAN_POINT('Ctrl Pts',(-0.655782055676547,-2.48549706819932,
7.60504883404085));
#12236=CARTESIAN_POINT('Ctrl Pts',(-0.488152229522925,-2.50642282845949,
7.39416068503242));
#12237=CARTESIAN_POINT('Ctrl Pts',(-0.17617063943151,-2.53326677800351,
7.24407668777915));
#12238=CARTESIAN_POINT('Ctrl Pts',(0.168881610443051,-2.56004874071718,
7.24418064291107));
#12239=CARTESIAN_POINT('Ctrl Pts',(0.479230965544757,-2.58677333437478,
7.39370222330362));
#12240=CARTESIAN_POINT('Ctrl Pts',(0.693414173896507,-2.61344224384572,
7.66242541074539));
#12241=CARTESIAN_POINT('Ctrl Pts',(0.769764263667122,-2.64005723004352,
7.99696854387048));
#12242=CARTESIAN_POINT('Ctrl Pts',(0.693335561872293,-2.66662311576071,
8.3304793629683));
#12243=CARTESIAN_POINT('Ctrl Pts',(0.456681051153885,-2.69608560261765,
8.62783081941731));
#12244=CARTESIAN_POINT('Ctrl Pts',(0.16924819913035,-2.7196091352219,8.7407546542504));
#12245=CARTESIAN_POINT('Ctrl Pts',(-0.0529090347140539,-2.73722886357395,
8.74031178383068));
#12246=CARTESIAN_POINT('Ctrl Pts',(-0.23576095072381,-2.75190456253053,
8.71294659686804));
#12247=CARTESIAN_POINT('Ctrl Pts',(-0.474181034064131,-2.77242751342201,
8.59809544867928));
#12248=CARTESIAN_POINT('Ctrl Pts',(-0.685755228804926,-2.79877927012082,
8.33265644851143));
#12249=CARTESIAN_POINT('Ctrl Pts',(-0.774362457417276,-2.82948181440773,
7.94678514096296));
#12250=CARTESIAN_POINT('Ctrl Pts',(-0.62102565384786,-2.86451451341815,
7.5070541202394));
#12251=CARTESIAN_POINT('Ctrl Pts',(-0.177411403127165,-2.90386624093258,
7.22859186809493));
#12252=CARTESIAN_POINT('Ctrl Pts',(0.341805275122635,-2.94316555019382,
7.28718194578695));
#12253=CARTESIAN_POINT('Ctrl Pts',(0.711089238372315,-2.98242344371321,
7.65669609347703));
#12254=CARTESIAN_POINT('Ctrl Pts',(0.759874955551073,-3.01511362277788,
8.08842693995537));
#12255=CARTESIAN_POINT('Ctrl Pts',(0.631394082076154,-3.04125498629743,
8.39617192670839));
#12256=CARTESIAN_POINT('Ctrl Pts',(0.446727094145398,-3.06303575794805,
8.60328587127767));
#12257=CARTESIAN_POINT('Ctrl Pts',(0.168447547207533,-3.08698931162158,
8.73726657609774));
#12258=CARTESIAN_POINT('Ctrl Pts',(-0.168284740868862,-3.11312097384991,
8.73735081104941));
#12259=CARTESIAN_POINT('Ctrl Pts',(-0.471770516529958,-3.13925157733386,
8.5911521718779));
#12260=CARTESIAN_POINT('Ctrl Pts',(-0.681876290605352,-3.16538945158193,
8.32788280407561));
#12261=CARTESIAN_POINT('Ctrl Pts',(-0.75687043959184,-3.19153241519703,
7.99933013384828));
#12262=CARTESIAN_POINT('Ctrl Pts',(-0.688110617431308,-3.21550770668684,
7.69802709281149));
#12263=CARTESIAN_POINT('Ctrl Pts',(-0.527102437271904,-3.23731354435981,
7.47155051476055));
#12264=CARTESIAN_POINT('Ctrl Pts',(-0.255247811551174,-3.26349398274227,
7.27779274208));
#12265=CARTESIAN_POINT('Ctrl Pts',(0.177152842785472,-3.29623830622227,
7.22824975845271));
#12266=CARTESIAN_POINT('Ctrl Pts',(0.620660945134379,-3.33559389149627,
7.50721088384051));
#12267=CARTESIAN_POINT('Ctrl Pts',(0.735928860988268,-3.36185737845845,
7.8361523880049));
#12268=CARTESIAN_POINT('Ctrl Pts',(0.735951464222257,-3.37501503233047,
8.0019910392312));
#12269=CARTESIAN_POINT('Ctrl Pts',(0.829757440060419,-2.26160662142564,
7.99511618081194));
#12270=CARTESIAN_POINT('Ctrl Pts',(0.829732011685375,-2.27640882444931,
8.18168267713667));
#12271=CARTESIAN_POINT('Ctrl Pts',(0.699816007409573,-2.30598791214416,
8.55221812941387));
#12272=CARTESIAN_POINT('Ctrl Pts',(0.201827204414,-2.35015821050548,8.86470616099201));
#12273=CARTESIAN_POINT('Ctrl Pts',(-0.379023488117868,-2.39415086067652,
8.798733952075));
#12274=CARTESIAN_POINT('Ctrl Pts',(-0.807163231352076,-2.43957549257121,
8.37081904005922));
#12275=CARTESIAN_POINT('Ctrl Pts',(-0.840454824876188,-2.47348909800905,
7.91591570873383));
#12276=CARTESIAN_POINT('Ctrl Pts',(-0.705987307445184,-2.50247231543482,
7.57601597628261));
#12277=CARTESIAN_POINT('Ctrl Pts',(-0.525755857322679,-2.52497039347374,
7.34930933428415));
#12278=CARTESIAN_POINT('Ctrl Pts',(-0.190564709372351,-2.55381055956905,
7.18809737406272));
#12279=CARTESIAN_POINT('Ctrl Pts',(0.179868561363044,-2.58256433966825,
7.18824648518451));
#12280=CARTESIAN_POINT('Ctrl Pts',(0.512742434807326,-2.61123160277901,
7.3486676190774));
#12281=CARTESIAN_POINT('Ctrl Pts',(0.742233225896921,-2.63981211857978,
7.63666503815448));
#12282=CARTESIAN_POINT('Ctrl Pts',(0.823917156000059,-2.66830610941488,
7.99481197794227));
#12283=CARTESIAN_POINT('Ctrl Pts',(0.742148744255773,-2.69671317878052,
8.35141437252788));
#12284=CARTESIAN_POINT('Ctrl Pts',(0.489351482775192,-2.72818096959852,
8.66894559809407));
#12285=CARTESIAN_POINT('Ctrl Pts',(0.182823382372039,-2.75326575186073,
8.78927701682514));
#12286=CARTESIAN_POINT('Ctrl Pts',(-0.0537740200675628,-2.77203170033953,
8.78879919988707));
#12287=CARTESIAN_POINT('Ctrl Pts',(-0.248418830469036,-2.78765413923565,
8.75966578777999));
#12288=CARTESIAN_POINT('Ctrl Pts',(-0.501950393695151,-2.80948215695733,
8.6374786190774));
#12289=CARTESIAN_POINT('Ctrl Pts',(-0.726531624311689,-2.83746139454138,
8.35561440545181));
#12290=CARTESIAN_POINT('Ctrl Pts',(-0.820370674170875,-2.8700064123799,
7.94658577453689));
#12291=CARTESIAN_POINT('Ctrl Pts',(-0.657979802162612,-2.90706403447766,
7.48157410220611));
#12292=CARTESIAN_POINT('Ctrl Pts',(-0.189982629638962,-2.9485699800761,
7.18813916684599));
#12293=CARTESIAN_POINT('Ctrl Pts',(0.355914283630534,-2.98989709841734,
7.2500307715348));
#12294=CARTESIAN_POINT('Ctrl Pts',(0.742747929313828,-3.03104923641469,
7.63753899362132));
#12295=CARTESIAN_POINT('Ctrl Pts',(0.793447036700908,-3.06520022873892,
8.08855426316809));
#12296=CARTESIAN_POINT('Ctrl Pts',(0.659538652208142,-3.09243881334936,
8.40914673502315));
#12297=CARTESIAN_POINT('Ctrl Pts',(0.4674503800378,-3.11509225286223,8.62451838266328));
#12298=CARTESIAN_POINT('Ctrl Pts',(0.178601860616001,-3.13995544254992,
8.76348553257992));
#12299=CARTESIAN_POINT('Ctrl Pts',(-0.169989036987309,-3.16700866084923,
8.76347040877462));
#12300=CARTESIAN_POINT('Ctrl Pts',(-0.483342670519688,-3.19399683667518,
8.61240741646133));
#12301=CARTESIAN_POINT('Ctrl Pts',(-0.699654697307745,-3.22091820440651,
8.34118976706614));
#12302=CARTESIAN_POINT('Ctrl Pts',(-0.776595267516835,-3.24777858249128,
8.00364839053361));
#12303=CARTESIAN_POINT('Ctrl Pts',(-0.706051258169142,-3.27234450691577,
7.69497590786256));
#12304=CARTESIAN_POINT('Ctrl Pts',(-0.541450566177014,-3.29463393432445,
7.46352675713963));
#12305=CARTESIAN_POINT('Ctrl Pts',(-0.264114921152119,-3.32133928901001,
7.2659407429079));
#12306=CARTESIAN_POINT('Ctrl Pts',(0.175653891720555,-3.35464280170236,
7.21584666351496));
#12307=CARTESIAN_POINT('Ctrl Pts',(0.624550632429727,-3.39449891025175,
7.49865340549804));
#12308=CARTESIAN_POINT('Ctrl Pts',(0.740598756530013,-3.42098439776615,
7.83036302208991));
#12309=CARTESIAN_POINT('Ctrl Pts',(0.740621508425407,-3.43422858948904,
7.99729239363825));
#12310=CARTESIAN_POINT('Ctrl Pts',(0.86707857137678,-2.21527214004116,7.99879744958048));
#12311=CARTESIAN_POINT('Ctrl Pts',(0.867052009824273,-2.23073398108044,
8.19367800248297));
#12312=CARTESIAN_POINT('Ctrl Pts',(0.731286147591186,-2.26168598382591,
8.58142473244992));
#12313=CARTESIAN_POINT('Ctrl Pts',(0.208931008692675,-2.30803255060304,
8.90953225625817));
#12314=CARTESIAN_POINT('Ctrl Pts',(-0.402279795131404,-2.35432607147985,
8.84040847995338));
#12315=CARTESIAN_POINT('Ctrl Pts',(-0.85419214733997,-2.40225297340794,
8.38916286237217));
#12316=CARTESIAN_POINT('Ctrl Pts',(-0.88965534661522,-2.4381319659943,7.90795747806708));
#12317=CARTESIAN_POINT('Ctrl Pts',(-0.747191693894078,-2.4688399396954,
7.54781745305364));
#12318=CARTESIAN_POINT('Ctrl Pts',(-0.556071742805826,-2.49270484793502,
7.30732995556476));
#12319=CARTESIAN_POINT('Ctrl Pts',(-0.200048697492744,-2.52334022091847,
7.13602410911045));
#12320=CARTESIAN_POINT('Ctrl Pts',(0.194018639288425,-2.55393045636901,
7.13611701708511));
#12321=CARTESIAN_POINT('Ctrl Pts',(0.548640567302356,-2.58446945367359,
7.3069515339409));
#12322=CARTESIAN_POINT('Ctrl Pts',(0.793472676065515,-2.61495596112549,
7.61410479143909));
#12323=CARTESIAN_POINT('Ctrl Pts',(0.880764541866717,-2.64538780695502,
7.99658056852376));
#12324=CARTESIAN_POINT('Ctrl Pts',(0.793387375209798,-2.67576077225686,
8.37786647565061));
#12325=CARTESIAN_POINT('Ctrl Pts',(0.522853213263504,-2.70944332490509,
8.71777142840022));
#12326=CARTESIAN_POINT('Ctrl Pts',(0.194405270094262,-2.73632442536312,
8.8467788012416));
#12327=CARTESIAN_POINT('Ctrl Pts',(-0.0593225760385914,-2.75644899867342,
8.84627081900103));
#12328=CARTESIAN_POINT('Ctrl Pts',(-0.26811681268387,-2.77320721193081,
8.81502223178674));
#12329=CARTESIAN_POINT('Ctrl Pts',(-0.540247683922515,-2.79663560807698,
8.68390627847152));
#12330=CARTESIAN_POINT('Ctrl Pts',(-0.78149729335789,-2.82668832932834,
8.38117208069794));
#12331=CARTESIAN_POINT('Ctrl Pts',(-0.882393815086409,-2.86166862077938,
7.94154547407333));
#12332=CARTESIAN_POINT('Ctrl Pts',(-0.707795934997192,-2.90152720543561,
7.44135040812137));
#12333=CARTESIAN_POINT('Ctrl Pts',(-0.204107195235052,-2.94620036140782,
7.12545965332791));
#12334=CARTESIAN_POINT('Ctrl Pts',(0.383742278004164,-2.99070111215732,
7.19206409213777));
#12335=CARTESIAN_POINT('Ctrl Pts',(0.800421419505439,-3.03502472007537,
7.60944125035824));
#12336=CARTESIAN_POINT('Ctrl Pts',(0.855035679658814,-3.0718098054969,8.0952640245661));
#12337=CARTESIAN_POINT('Ctrl Pts',(0.710808338022248,-3.10114549328222,
8.44055327044642));
#12338=CARTESIAN_POINT('Ctrl Pts',(0.503947744187646,-3.12554011221735,
8.67248640703811));
#12339=CARTESIAN_POINT('Ctrl Pts',(0.192957910284852,-3.1523069335416,8.82209610703405));
#12340=CARTESIAN_POINT('Ctrl Pts',(-0.182227420528306,-3.18142312386516,
8.82206702034478));
#12341=CARTESIAN_POINT('Ctrl Pts',(-0.519316204583526,-3.2104536203229,
8.65954066193778));
#12342=CARTESIAN_POINT('Ctrl Pts',(-0.751885348749804,-3.23939925187631,
8.36790792232583));
#12343=CARTESIAN_POINT('Ctrl Pts',(-0.834531785156997,-3.26825784301778,
8.00521528728933));
#12344=CARTESIAN_POINT('Ctrl Pts',(-0.758762890055745,-3.29463265406983,
7.67379560957547));
#12345=CARTESIAN_POINT('Ctrl Pts',(-0.582145976295626,-3.31854651420027,
7.42547621523144));
#12346=CARTESIAN_POINT('Ctrl Pts',(-0.284767910361057,-3.3471788646333,
7.21363048066223));
#12347=CARTESIAN_POINT('Ctrl Pts',(0.186219878216593,-3.38284229741198,
7.16011863942536));
#12348=CARTESIAN_POINT('Ctrl Pts',(0.666069785790777,-3.42545036202905,
7.46260932525095));
#12349=CARTESIAN_POINT('Ctrl Pts',(0.789761191020466,-3.45371486538175,
7.8167106365808));
#12350=CARTESIAN_POINT('Ctrl Pts',(0.789785439415121,-3.46783018993909,
7.99461973868823));
#12351=CARTESIAN_POINT('Ctrl Pts',(0.853613778380816,-2.15732131048097,
8.00339343853682));
#12352=CARTESIAN_POINT('Ctrl Pts',(0.853587606604479,-2.17255625750892,
8.19541422653387));
#12353=CARTESIAN_POINT('Ctrl Pts',(0.71993526562251,-2.20307513036369,8.57788731388851));
#12354=CARTESIAN_POINT('Ctrl Pts',(0.202998077757662,-2.24895826646226,
8.90308049625081));
#12355=CARTESIAN_POINT('Ctrl Pts',(-0.404350822674032,-2.29494956399607,
8.83473441415818));
#12356=CARTESIAN_POINT('Ctrl Pts',(-0.855322089232105,-2.34274179079025,
8.38500627260658));
#12357=CARTESIAN_POINT('Ctrl Pts',(-0.891159898667268,-2.3786574478564,
7.90325459408232));
#12358=CARTESIAN_POINT('Ctrl Pts',(-0.748187122836472,-2.40947785315607,
7.54177066796142));
#12359=CARTESIAN_POINT('Ctrl Pts',(-0.556127946781633,-2.43346472037247,
7.29998095570304));
#12360=CARTESIAN_POINT('Ctrl Pts',(-0.197400708727537,-2.46433665913889,
7.1272421567771));
#12361=CARTESIAN_POINT('Ctrl Pts',(0.200669460267103,-2.4952342052595,7.12723282118374));
#12362=CARTESIAN_POINT('Ctrl Pts',(0.559810871311599,-2.52615645882231,
7.30012245677509));
#12363=CARTESIAN_POINT('Ctrl Pts',(0.808408390951575,-2.55709970891155,
7.61183546841623));
#12364=CARTESIAN_POINT('Ctrl Pts',(0.897329380531666,-2.58806086349922,
8.00097004624504));
#12365=CARTESIAN_POINT('Ctrl Pts',(0.808306642551815,-2.61903782660728,
8.38987609029684));
#12366=CARTESIAN_POINT('Ctrl Pts',(0.531836448053288,-2.65346946876861,
8.73743082896215));
#12367=CARTESIAN_POINT('Ctrl Pts',(0.195204243964366,-2.68102443097052,
8.86982140892509));
#12368=CARTESIAN_POINT('Ctrl Pts',(-0.0654014761015361,-2.70169345944525,
8.8693080479456));
#12369=CARTESIAN_POINT('Ctrl Pts',(-0.28001061760865,-2.71891842965623,
8.83719397053499));
#12370=CARTESIAN_POINT('Ctrl Pts',(-0.56017691686546,-2.74303440031375,
8.70229225968454));
#12371=CARTESIAN_POINT('Ctrl Pts',(-0.809160087931685,-2.77404089873971,
8.39000815585855));
#12372=CARTESIAN_POINT('Ctrl Pts',(-0.913602970950101,-2.81021106185289,
7.93545491025926));
#12373=CARTESIAN_POINT('Ctrl Pts',(-0.732844719291178,-2.85153775103447,
7.41673989523743));
#12374=CARTESIAN_POINT('Ctrl Pts',(-0.209092138228919,-2.898005510644,7.08787736303838));
#12375=CARTESIAN_POINT('Ctrl Pts',(0.404314566935514,-2.94443832383181,
7.15706703724753));
#12376=CARTESIAN_POINT('Ctrl Pts',(0.840611098505371,-2.99082585871325,
7.59366406143764));
#12377=CARTESIAN_POINT('Ctrl Pts',(0.898167561855067,-3.0294358538606,8.10354953547171));
#12378=CARTESIAN_POINT('Ctrl Pts',(0.746510298453132,-3.06029121684836,
8.4667497767436));
#12379=CARTESIAN_POINT('Ctrl Pts',(0.528670012322939,-3.08598436655093,
8.71104238802412));
#12380=CARTESIAN_POINT('Ctrl Pts',(0.200651339320336,-3.11422060483273,
8.86892278377001));
#12381=CARTESIAN_POINT('Ctrl Pts',(-0.195786982033943,-3.14498685758523,
8.86896376428506));
#12382=CARTESIAN_POINT('Ctrl Pts',(-0.552599640454179,-3.17571518690325,
8.69700649395508));
#12383=CARTESIAN_POINT('Ctrl Pts',(-0.799192405052644,-3.20640067964169,
8.38789335444557));
#12384=CARTESIAN_POINT('Ctrl Pts',(-0.887002523210114,-3.23704301100247,
8.00282800313923));
#12385=CARTESIAN_POINT('Ctrl Pts',(-0.806491468029696,-3.2650882512832,
7.65042392555724));
#12386=CARTESIAN_POINT('Ctrl Pts',(-0.6184882410522,-3.29054770478482,7.38606022980516));
#12387=CARTESIAN_POINT('Ctrl Pts',(-0.301617462444111,-3.32105973226801,
7.16028129179456));
#12388=CARTESIAN_POINT('Ctrl Pts',(0.201027370363033,-3.3591287320595,7.10307029008688));
#12389=CARTESIAN_POINT('Ctrl Pts',(0.714123794960093,-3.40467760024813,
7.42624743346387));
#12390=CARTESIAN_POINT('Ctrl Pts',(0.846710623234168,-3.43496022264899,
7.80554292001516));
#12391=CARTESIAN_POINT('Ctrl Pts',(0.846736584716904,-3.45007275937647,
7.99602085262167));
#12392=CARTESIAN_POINT('Ctrl Pts',(0.817951311059339,-2.14018795858917,
8.00474793958371));
#12393=CARTESIAN_POINT('Ctrl Pts',(0.817926216049528,-2.15479610517542,
8.18886855474053));
#12394=CARTESIAN_POINT('Ctrl Pts',(0.689817303447149,-2.18405877779726,
8.55560183955968));
#12395=CARTESIAN_POINT('Ctrl Pts',(0.19347377106145,-2.22812384223798,8.86803409341903));
#12396=CARTESIAN_POINT('Ctrl Pts',(-0.390624346224737,-2.27235269475253,
8.80243528497531));
#12397=CARTESIAN_POINT('Ctrl Pts',(-0.825118707115923,-2.3183864962394,
8.36940838838631));
#12398=CARTESIAN_POINT('Ctrl Pts',(-0.859860802914712,-2.35303977428868,
7.9046020627869));
#12399=CARTESIAN_POINT('Ctrl Pts',(-0.721763577837354,-2.38281053702234,
7.55541942075108));
#12400=CARTESIAN_POINT('Ctrl Pts',(-0.536133762339803,-2.40599896833622,
7.32165570099066));
#12401=CARTESIAN_POINT('Ctrl Pts',(-0.18895749473576,-2.43587876194045,
7.15441590182363));
#12402=CARTESIAN_POINT('Ctrl Pts',(0.196802128379297,-2.46582051078235,
7.15434610219188));
#12403=CARTESIAN_POINT('Ctrl Pts',(0.545307786053435,-2.49582411881007,
7.32204685195694));
#12404=CARTESIAN_POINT('Ctrl Pts',(0.786887979130198,-2.52588746642215,
7.62486140910485));
#12405=CARTESIAN_POINT('Ctrl Pts',(0.873463361515396,-2.55600774488533,
8.00342516000178));
#12406=CARTESIAN_POINT('Ctrl Pts',(0.78679367211852,-2.58618568236755,8.38231958055917));
#12407=CARTESIAN_POINT('Ctrl Pts',(0.517143884962038,-2.61977459658829,
8.72142638757352));
#12408=CARTESIAN_POINT('Ctrl Pts',(0.188227088153933,-2.64670029064388,
8.85088945134281));
#12409=CARTESIAN_POINT('Ctrl Pts',(-0.0667518101348738,-2.6669222358181,
8.85039427757092));
#12410=CARTESIAN_POINT('Ctrl Pts',(-0.276825487921848,-2.68378301119882,
8.81896286031109));
#12411=CARTESIAN_POINT('Ctrl Pts',(-0.551354493616545,-2.7074097040812,
8.68683667774742));
#12412=CARTESIAN_POINT('Ctrl Pts',(-0.795733091743474,-2.73783532831967,
8.38043509041218));
#12413=CARTESIAN_POINT('Ctrl Pts',(-0.898456345943392,-2.77338063567163,
7.93373612144092));
#12414=CARTESIAN_POINT('Ctrl Pts',(-0.720680695041125,-2.81406632664805,
7.42293130178022));
#12415=CARTESIAN_POINT('Ctrl Pts',(-0.203901168868501,-2.85992243385813,
7.09814633450196));
#12416=CARTESIAN_POINT('Ctrl Pts',(0.402960792325747,-2.90585094023315,
7.16634457332539));
#12417=CARTESIAN_POINT('Ctrl Pts',(0.835793473763965,-2.95184458747716,
7.59911373795158));
#12418=CARTESIAN_POINT('Ctrl Pts',(0.893222610079682,-2.99022150713542,
8.1059459436348));
#12419=CARTESIAN_POINT('Ctrl Pts',(0.742230061053853,-3.02094600804868,
8.46767578677156));
#12420=CARTESIAN_POINT('Ctrl Pts',(0.525050043132394,-3.04656270442428,
8.7112819718791));
#12421=CARTESIAN_POINT('Ctrl Pts',(0.197561468846462,-3.07475163348297,
8.86898675520401));
#12422=CARTESIAN_POINT('Ctrl Pts',(-0.198942516484079,-3.10552114011045,
8.86910705024245));
#12423=CARTESIAN_POINT('Ctrl Pts',(-0.556404604870121,-3.13629694361956,
8.69691854995843));
#12424=CARTESIAN_POINT('Ctrl Pts',(-0.803908575128165,-3.16708632463838,
8.38679365490788));
#12425=CARTESIAN_POINT('Ctrl Pts',(-0.892230210331149,-3.19787639573897,
7.99981674999116));
#12426=CARTESIAN_POINT('Ctrl Pts',(-0.811254302996053,-3.22610486728836,
7.64504873212211));
#12427=CARTESIAN_POINT('Ctrl Pts',(-0.621751910267926,-3.25176808988285,
7.37851925540117));
#12428=CARTESIAN_POINT('Ctrl Pts',(-0.301953097190216,-3.28256284856841,
7.15059667963661));
#12429=CARTESIAN_POINT('Ctrl Pts',(0.206209630770826,-3.32104498703397,
7.092565584774));
#12430=CARTESIAN_POINT('Ctrl Pts',(0.726383216812123,-3.36720427357741,
7.41989946778657));
#12431=CARTESIAN_POINT('Ctrl Pts',(0.861157216643285,-3.39796397231344,
7.80525499237318));
#12432=CARTESIAN_POINT('Ctrl Pts',(0.861183614424057,-3.41333048413908,
7.99893401904505));
#12433=CARTESIAN_POINT('Ctrl Pts',(0.799999353205571,-2.14018795858917,
8.00474549279328));
#12434=CARTESIAN_POINT('Ctrl Pts',(0.799974799734663,-2.15448086801293,
8.18489286877592));
#12435=CARTESIAN_POINT('Ctrl Pts',(0.674665007466417,-2.18310389914977,
8.54360793631645));
#12436=CARTESIAN_POINT('Ctrl Pts',(0.189057319427946,-2.22621797906703,
8.84931316013818));
#12437=CARTESIAN_POINT('Ctrl Pts',(-0.382526459311769,-2.26949883233014,
8.78512361823764));
#12438=CARTESIAN_POINT('Ctrl Pts',(-0.807840639236961,-2.31455899583364,
8.36128354752488));
#12439=CARTESIAN_POINT('Ctrl Pts',(-0.841884630553248,-2.34849059789531,
7.90616153590567));
#12440=CARTESIAN_POINT('Ctrl Pts',(-0.706633312481697,-2.3776482221266,
7.56417102566761));
#12441=CARTESIAN_POINT('Ctrl Pts',(-0.524797421299121,-2.40036397277687,
7.33517763260607));
#12442=CARTESIAN_POINT('Ctrl Pts',(-0.184623097405697,-2.42964203470304,
7.17129916558269));
#12443=CARTESIAN_POINT('Ctrl Pts',(0.193484153574259,-2.4589910981866,7.17122122775637));
#12444=CARTESIAN_POINT('Ctrl Pts',(0.53519122257586,-2.48841027946974,7.33563982396839));
#12445=CARTESIAN_POINT('Ctrl Pts',(0.772150285550503,-2.51789845810207,
7.63264106317873));
#12446=CARTESIAN_POINT('Ctrl Pts',(0.857109363647141,-2.54745448449862,
8.00408762003218));
#12447=CARTESIAN_POINT('Ctrl Pts',(0.772052203859602,-2.5770771143395,8.37600483173473));
#12448=CARTESIAN_POINT('Ctrl Pts',(0.507269008134946,-2.61006365580992,
8.70902087610833));
#12449=CARTESIAN_POINT('Ctrl Pts',(0.184121132841334,-2.63651910824196,
8.83624322508014));
#12450=CARTESIAN_POINT('Ctrl Pts',(-0.066489483803979,-2.65639505342702,
8.83575881359142));
#12451=CARTESIAN_POINT('Ctrl Pts',(-0.272993262404685,-2.67296969383809,
8.80486180272118));
#12452=CARTESIAN_POINT('Ctrl Pts',(-0.542963798600168,-2.69620569938568,
8.6749478571166));
#12453=CARTESIAN_POINT('Ctrl Pts',(-0.783400610994973,-2.72613969346878,
8.3735180635455));
#12454=CARTESIAN_POINT('Ctrl Pts',(-0.884539863210645,-2.76112964475965,
7.93383176138089));
#12455=CARTESIAN_POINT('Ctrl Pts',(-0.709496036003296,-2.80121083689286,
7.43066574821048));
#12456=CARTESIAN_POINT('Ctrl Pts',(-0.200096069822599,-2.84642092016874,
7.11042023888795));
#12457=CARTESIAN_POINT('Ctrl Pts',(0.398680163779428,-2.89174303462223,
7.17762409038781));
#12458=CARTESIAN_POINT('Ctrl Pts',(0.826194257186495,-2.93717015873569,
7.60494403903258));
#12459=CARTESIAN_POINT('Ctrl Pts',(0.883028763967666,-2.97510749619044,
8.10591734828594));
#12460=CARTESIAN_POINT('Ctrl Pts',(0.733685094600885,-3.00550240345549,
8.46374186218363));
#12461=CARTESIAN_POINT('Ctrl Pts',(0.518762431301621,-3.03085542203816,
8.70482943573385));
#12462=CARTESIAN_POINT('Ctrl Pts',(0.194479876070813,-3.05877306117867,
8.86101946641206));
#12463=CARTESIAN_POINT('Ctrl Pts',(-0.198398854087579,-3.08926279897463,
8.86116295997746));
#12464=CARTESIAN_POINT('Ctrl Pts',(-0.552866770740287,-3.11978430147565,
8.69045288806385));
#12465=CARTESIAN_POINT('Ctrl Pts',(-0.798459570530803,-3.15033499607393,
8.38276097552609));
#12466=CARTESIAN_POINT('Ctrl Pts',(-0.886189886223361,-3.18091257250085,
7.9985222617957));
#12467=CARTESIAN_POINT('Ctrl Pts',(-0.805754444707439,-3.20896404488721,
7.64600910454789));
#12468=CARTESIAN_POINT('Ctrl Pts',(-0.617356025266483,-3.23448146889928,
7.38101130632405));
#12469=CARTESIAN_POINT('Ctrl Pts',(-0.299249903140631,-3.2651162608211,
7.15427322620025));
#12470=CARTESIAN_POINT('Ctrl Pts',(0.20669102063405,-3.30343842772452,7.09641469177514));
#12471=CARTESIAN_POINT('Ctrl Pts',(0.72520383869486,-3.34944736574065,7.4225450742071));
#12472=CARTESIAN_POINT('Ctrl Pts',(0.859802571238952,-3.38014846116659,
7.80703861326121));
#12473=CARTESIAN_POINT('Ctrl Pts',(0.859828918911975,-3.39548580458109,
8.00035000220606));
#12474=CARTESIAN_POINT('Ctrl Pts',(0.753146974179187,-2.1619943924303,8.27380160983776));
#12475=CARTESIAN_POINT('Ctrl Pts',(0.723482246295192,-2.16903452865882,
8.35718646810225));
#12476=CARTESIAN_POINT('Ctrl Pts',(0.680269466184233,-2.17608055625528,
8.43571695267455));
#12477=CARTESIAN_POINT('Ctrl Pts',(0.6250578408604,-2.18313382135177,8.50488004006827));
#12478=CARTESIAN_POINT('Ctrl Pts',(0.51279577812026,-2.19747525912219,8.64550967759036));
#12479=CARTESIAN_POINT('Ctrl Pts',(0.350926548774103,-2.21184661909461,
8.74741141886427));
#12480=CARTESIAN_POINT('Ctrl Pts',(0.174727970977739,-2.22624577462467,
8.7876640325178));
#12481=CARTESIAN_POINT('Ctrl Pts',(-0.00147060681862579,-2.24064493015473,
8.82791664617134));
#12482=CARTESIAN_POINT('Ctrl Pts',(-0.191998533065198,-2.25507188124244,
8.80652013220449));
#12483=CARTESIAN_POINT('Ctrl Pts',(-0.355616560819318,-2.26952716877793,
8.72770472099937));
#12484=CARTESIAN_POINT('Ctrl Pts',(-0.519234588573438,-2.28398245631341,
8.64888930979425));
#12485=CARTESIAN_POINT('Ctrl Pts',(-0.655942717835107,-2.29846608029668,
8.51265500135086));
#12486=CARTESIAN_POINT('Ctrl Pts',(-0.734805551021998,-2.31297741063122,
8.34855954342037));
#12487=CARTESIAN_POINT('Ctrl Pts',(-0.822430921229655,-2.32910111100293,
8.16623125683093));
#12488=CARTESIAN_POINT('Ctrl Pts',(-0.838642345665982,-2.34525901674658,
7.94950648939321));
#12489=CARTESIAN_POINT('Ctrl Pts',(-0.778727898779652,-2.36145090114427,
7.75505675489523));
#12490=CARTESIAN_POINT('Ctrl Pts',(-0.766745009402386,-2.36468927802381,
7.71616680799563));
#12491=CARTESIAN_POINT('Ctrl Pts',(-0.751717085172214,-2.3679290140495,
7.67816786241363));
#12492=CARTESIAN_POINT('Ctrl Pts',(-0.733952003028779,-2.37117009287772,
7.64149031776064));
#12493=CARTESIAN_POINT('Ctrl Pts',(-0.680656756598472,-2.38089332936235,
7.53145768380167));
#12494=CARTESIAN_POINT('Ctrl Pts',(-0.602727088948797,-2.39062865106961,
7.43331765820387));
#12495=CARTESIAN_POINT('Ctrl Pts',(-0.507066534475055,-2.40037598891093,
7.35693456756774));
#12496=CARTESIAN_POINT('Ctrl Pts',(-0.411405980001313,-2.41012332675226,
7.28055147693161));
#12497=CARTESIAN_POINT('Ctrl Pts',(-0.298014538703504,-2.41988268072765,
7.22592532125715));
#12498=CARTESIAN_POINT('Ctrl Pts',(-0.178300942891275,-2.42965386829594,
7.1985992537822));
#12499=CARTESIAN_POINT('Ctrl Pts',(-0.0585873470790449,-2.43942505586423,
7.17127318630725));
#12500=CARTESIAN_POINT('Ctrl Pts',(0.0674484032476069,-2.44920807702541,
7.17124720703181));
#12501=CARTESIAN_POINT('Ctrl Pts',(0.187417456577866,-2.45900278448653,
7.19863731676276));
#12502=CARTESIAN_POINT('Ctrl Pts',(0.307386509908125,-2.46879749194765,
7.22602742649371));
#12503=CARTESIAN_POINT('Ctrl Pts',(0.421288866241992,-2.4786038857087,7.28083362523105));
#12504=CARTESIAN_POINT('Ctrl Pts',(0.517733221571367,-2.48842177902794,
7.35773693113477));
#12505=CARTESIAN_POINT('Ctrl Pts',(0.61417757690074,-2.49823967234718,7.4346402370385));
#12506=CARTESIAN_POINT('Ctrl Pts',(0.693163931225622,-2.50806906522463,
7.53364065010862));
#12507=CARTESIAN_POINT('Ctrl Pts',(0.746816954737502,-2.51790976606277,
7.64504861611925));
#12508=CARTESIAN_POINT('Ctrl Pts',(0.800469978249382,-2.52775046690092,
7.75645658212988));
#12509=CARTESIAN_POINT('Ctrl Pts',(0.828789670948262,-2.53760247569977,
7.88027210108103));
#12510=CARTESIAN_POINT('Ctrl Pts',(0.828773323999778,-2.54746558507267,
8.00416606250703));
#12511=CARTESIAN_POINT('Ctrl Pts',(0.828756977051295,-2.55732869444558,
8.12806002393303));
#12512=CARTESIAN_POINT('Ctrl Pts',(0.800404590455449,-2.56720290439254,
8.25203242783388));
#12513=CARTESIAN_POINT('Ctrl Pts',(0.746510917798827,-2.57708799058658,
8.36397103644034));
#12514=CARTESIAN_POINT('Ctrl Pts',(0.692617245142206,-2.58697307678063,
8.47590964504681));
#12515=CARTESIAN_POINT('Ctrl Pts',(0.613182286424809,-2.59686903922175,
8.57581445835889));
#12516=CARTESIAN_POINT('Ctrl Pts',(0.515856401485537,-2.60677564404326,
8.65334937205055));
#12517=CARTESIAN_POINT('Ctrl Pts',(0.386088554899842,-2.61998445047194,
8.75672925697275));
#12518=CARTESIAN_POINT('Ctrl Pts',(0.224514617253036,-2.63321217668796,
8.82034043145866));
#12519=CARTESIAN_POINT('Ctrl Pts',(0.0585408341795072,-2.64645822602986,
8.83280431356186));
#12520=CARTESIAN_POINT('Ctrl Pts',(0.0170473884111253,-2.64976973836533,
8.83592028408766));
#12521=CARTESIAN_POINT('Ctrl Pts',(-0.0247210476964266,-2.65308239589618,
8.83583954883954));
#12522=CARTESIAN_POINT('Ctrl Pts',(-0.0662556436102732,-2.6563961887027,
8.83270948012845));
#12523=CARTESIAN_POINT('Ctrl Pts',(-0.10779023952412,-2.65970998150923,
8.82957941141737));
#12524=CARTESIAN_POINT('Ctrl Pts',(-0.149090995244261,-2.66302490959145,
8.82340000924332));
#12525=CARTESIAN_POINT('Ctrl Pts',(-0.189708366898492,-2.66634096299409,
8.81412567384119));
#12526=CARTESIAN_POINT('Ctrl Pts',(-0.311560481861183,-2.67628912320203,
8.78630266763481));
#12527=CARTESIAN_POINT('Ctrl Pts',(-0.427262140230675,-2.68624741129386,
8.73062526237571));
#12528=CARTESIAN_POINT('Ctrl Pts',(-0.525185771481222,-2.69621555435362,
8.65254826081764));
#12529=CARTESIAN_POINT('Ctrl Pts',(-0.623109402731769,-2.70618369741338,
8.57447125925957));
#12530=CARTESIAN_POINT('Ctrl Pts',(-0.703255006863371,-2.71616169544108,
8.47399466140254));
#12531=CARTESIAN_POINT('Ctrl Pts',(-0.757776273531411,-2.72614925892505,
8.36094403359336));
#12532=CARTESIAN_POINT('Ctrl Pts',(-0.81229754019945,-2.73613682240903,
8.24789340578418));
#12533=CARTESIAN_POINT('Ctrl Pts',(-0.841194469403928,-2.74613395134928,
8.12226874802287));
#12534=CARTESIAN_POINT('Ctrl Pts',(-0.84102824420588,-2.75614034792675,
7.99657735204903));
#12535=CARTESIAN_POINT('Ctrl Pts',(-0.840778906408808,-2.77114994279295,
7.80804025808828));
#12536=CARTESIAN_POINT('Ctrl Pts',(-0.775137471206052,-2.7861803898429,
7.61935300314938));
#12537=CARTESIAN_POINT('Ctrl Pts',(-0.657416759241225,-2.8012306272472,
7.47163512412617));
#12538=CARTESIAN_POINT('Ctrl Pts',(-0.539696047276397,-2.81628086465149,
7.32391724510297));
#12539=CARTESIAN_POINT('Ctrl Pts',(-0.369896058549498,-2.83135089241011,
7.21716874199546));
#12540=CARTESIAN_POINT('Ctrl Pts',(-0.185200025252378,-2.84643959203168,
7.17499513235835));
#12541=CARTESIAN_POINT('Ctrl Pts',(-0.000503991955257244,-2.86152829165324,
7.13282152272124));
#12542=CARTESIAN_POINT('Ctrl Pts',(0.199088085912085,-2.87663566313774,
7.15522280655453));
#12543=CARTESIAN_POINT('Ctrl Pts',(0.370136473746934,-2.89176053623223,
7.23764343991196));
#12544=CARTESIAN_POINT('Ctrl Pts',(0.541184861581783,-2.90688540932672,
7.3200640732694));
#12545=CARTESIAN_POINT('Ctrl Pts',(0.683689559384138,-2.92202778403121,
7.46250405615099));
#12546=CARTESIAN_POINT('Ctrl Pts',(0.766308809641551,-2.9371864388744,7.63391870944245));
#12547=CARTESIAN_POINT('Ctrl Pts',(0.848928059898963,-2.95234509371759,
7.80533336273392));
#12548=CARTESIAN_POINT('Ctrl Pts',(0.871661862611432,-2.96752002869949,
8.00572268643527));
#12549=CARTESIAN_POINT('Ctrl Pts',(0.829458573726661,-2.98270997611514,
8.19179396563495));
#12550=CARTESIAN_POINT('Ctrl Pts',(0.808356929284276,-2.99030494982297,
8.28482960523479));
#12551=CARTESIAN_POINT('Ctrl Pts',(0.77102101194258,-2.99790367663923,8.37428573370921));
#12552=CARTESIAN_POINT('Ctrl Pts',(0.720114653776843,-3.00550599283476,
8.45517693397895));
#12553=CARTESIAN_POINT('Ctrl Pts',(0.669208295611106,-3.01310830903029,
8.5360681342487));
#12554=CARTESIAN_POINT('Ctrl Pts',(0.604731496621327,-3.02071421460509,
8.60839440631376));
#12555=CARTESIAN_POINT('Ctrl Pts',(0.529984455678112,-3.02832354704088,
8.66797968224839));
#12556=CARTESIAN_POINT('Ctrl Pts',(0.430321734420493,-3.03846932362193,
8.7474267168279));
#12557=CARTESIAN_POINT('Ctrl Pts',(0.312400805245652,-3.0486211924003,8.80422309161998));
#12558=CARTESIAN_POINT('Ctrl Pts',(0.187960552298501,-3.05877874975548,
8.83264519461025));
#12559=CARTESIAN_POINT('Ctrl Pts',(0.0635202993513489,-3.06893630711065,
8.86106729760052));
#12560=CARTESIAN_POINT('Ctrl Pts',(-0.0674392773681153,-3.07909955304264,
8.86111512878899));
#12561=CARTESIAN_POINT('Ctrl Pts',(-0.191997051836632,-3.08926809309214,
8.83268736573095));
#12562=CARTESIAN_POINT('Ctrl Pts',(-0.316554826305149,-3.09943663314163,
8.80425960267292));
#12563=CARTESIAN_POINT('Ctrl Pts',(-0.434710798522717,-3.10961046730864,
8.74735624536838));
#12564=CARTESIAN_POINT('Ctrl Pts',(-0.534720917929921,-3.11978916682519,
8.66762258129316));
#12565=CARTESIAN_POINT('Ctrl Pts',(-0.634731037337125,-3.12996786634175,
8.58788891721793));
#12566=CARTESIAN_POINT('Ctrl Pts',(-0.716595303933964,-3.14015143120784,
8.48532494637201));
#12567=CARTESIAN_POINT('Ctrl Pts',(-0.772149156514476,-3.1503394763787,
8.37000317532732));
#12568=CARTESIAN_POINT('Ctrl Pts',(-0.827703009094989,-3.16052752154957,
8.25468140428263));
#12569=CARTESIAN_POINT('Ctrl Pts',(-0.856946447659175,-3.17072004702521,
8.12660183303916));
#12570=CARTESIAN_POINT('Ctrl Pts',(-0.8569435412111,-3.18091657746964,7.99846874609965));
#12571=CARTESIAN_POINT('Ctrl Pts',(-0.856940634763026,-3.19111310791407,
7.87033565916013));
#12572=CARTESIAN_POINT('Ctrl Pts',(-0.82769138330269,-3.20131364332729,
7.74214905652457));
#12573=CARTESIAN_POINT('Ctrl Pts',(-0.772093493947471,-3.21151785542143,
7.62664101580102));
#12574=CARTESIAN_POINT('Ctrl Pts',(-0.730395076931056,-3.21917101449204,
7.54000998525836));
#12575=CARTESIAN_POINT('Ctrl Pts',(-0.67387555109877,-3.22682624169566,
7.4605106457912));
#12576=CARTESIAN_POINT('Ctrl Pts',(-0.605852522916895,-3.2344832042877,
7.39241871604215));
#12577=CARTESIAN_POINT('Ctrl Pts',(-0.53782949473502,-3.24214016687973,
7.3243267862931));
#12578=CARTESIAN_POINT('Ctrl Pts',(-0.458302964203557,-3.24979886486019,
7.26764226626215));
#12579=CARTESIAN_POINT('Ctrl Pts',(-0.37155588226427,-3.25745947464072,
7.22599535061318));
#12580=CARTESIAN_POINT('Ctrl Pts',(-0.198061718385695,-3.27278069420178,
7.14270151931523));
#12581=CARTESIAN_POINT('Ctrl Pts',(0.00431465112417784,-3.28810956096315,
7.11955810554519));
#12582=CARTESIAN_POINT('Ctrl Pts',(0.191921638889249,-3.30344215067986,
7.16234146239883));
#12583=CARTESIAN_POINT('Ctrl Pts',(0.37952862665432,-3.31877474039656,7.20512481925246));
#12584=CARTESIAN_POINT('Ctrl Pts',(0.55236623267459,-3.33411105306861,7.31383494672978));
#12585=CARTESIAN_POINT('Ctrl Pts',(0.672434718820748,-3.34945448326111,
7.46431339523197));
#12586=CARTESIAN_POINT('Ctrl Pts',(0.780125650037461,-3.36321619824999,
7.59927940311118));
#12587=CARTESIAN_POINT('Ctrl Pts',(0.845366351460771,-3.37698363894322,
7.76784602494453));
#12588=CARTESIAN_POINT('Ctrl Pts',(0.857691923859112,-3.39074214267724,
7.9406445962268));
#14416=UNCERTAINTY_MEASURE_WITH_UNIT(LENGTH_MEASURE(0.001),#14513,
'DISTANCE_ACCURACY_VALUE',
'Maximum model space distance between geometric entities at asserted c
onnectivities');
#14455=UNCERTAINTY_MEASURE_WITH_UNIT(LENGTH_MEASURE(0.001),#14513,
'DISTANCE_ACCURACY_VALUE',
'Maximum model space distance between geometric entities at asserted c
onnectivities');
#14473=(
GEOMETRIC_REPRESENTATION_CONTEXT(3)
GLOBAL_UNCERTAINTY_ASSIGNED_CONTEXT((#14416))
GLOBAL_UNIT_ASSIGNED_CONTEXT((#14513,#14515,#14516))
REPRESENTATION_CONTEXT('','3D')
);
#14512=(
GEOMETRIC_REPRESENTATION_CONTEXT(3)
GLOBAL_UNCERTAINTY_ASSIGNED_CONTEXT((#14455))
GLOBAL_UNIT_ASSIGNED_CONTEXT((#14513,#14515,#14516))
REPRESENTATION_CONTEXT('','3D')
);
#14513=(
LENGTH_UNIT()
NAMED_UNIT(*)
SI_UNIT(.CENTI.,.METRE.)
);
#14515=(
NAMED_UNIT(*)
PLANE_ANGLE_UNIT()
SI_UNIT($,.RADIAN.)
);
#14516=(
NAMED_UNIT(*)
SI_UNIT($,.STERADIAN.)
SOLID_ANGLE_UNIT()
);
#14534=SHAPE_DEFINITION_REPRESENTATION(#14590,#14758);
#14590=PRODUCT_DEFINITION_SHAPE('',$,#14815);
#14758=SHAPE_REPRESENTATION('',(#8168),#14473);
#14797=PRODUCT_DEFINITION_CONTEXT('part definition',#14967,'design');
#14815=PRODUCT_DEFINITION('Installed torsion spring',
'Installed torsion spring',#14871,#14797);
#14871=PRODUCT_DEFINITION_FORMATION('',$,#14986);
#14967=APPLICATION_CONTEXT(
'Core Data for Automotive Mechanical Design Process');
#14968=PRODUCT_CONTEXT('part definition',#14967,'mechanical');
#14986=PRODUCT('Installed torsion spring','Installed torsion spring',
'Installed torsion spring',(#14968));
#15081=COLOUR_RGB('Grey',0.48,0.52,0.57);
#15082=FILL_AREA_STYLE_COLOUR('',#15081);
#15083=FILL_AREA_STYLE('',(#15082));
#15084=SURFACE_STYLE_FILL_AREA(#15083);
#15085=SURFACE_SIDE_STYLE('',(#15084));
#15086=SURFACE_STYLE_USAGE(.BOTH.,#15085);
#15087=PRESENTATION_STYLE_ASSIGNMENT((#15086));
ENDSEC;
END-ISO-10303-21;
